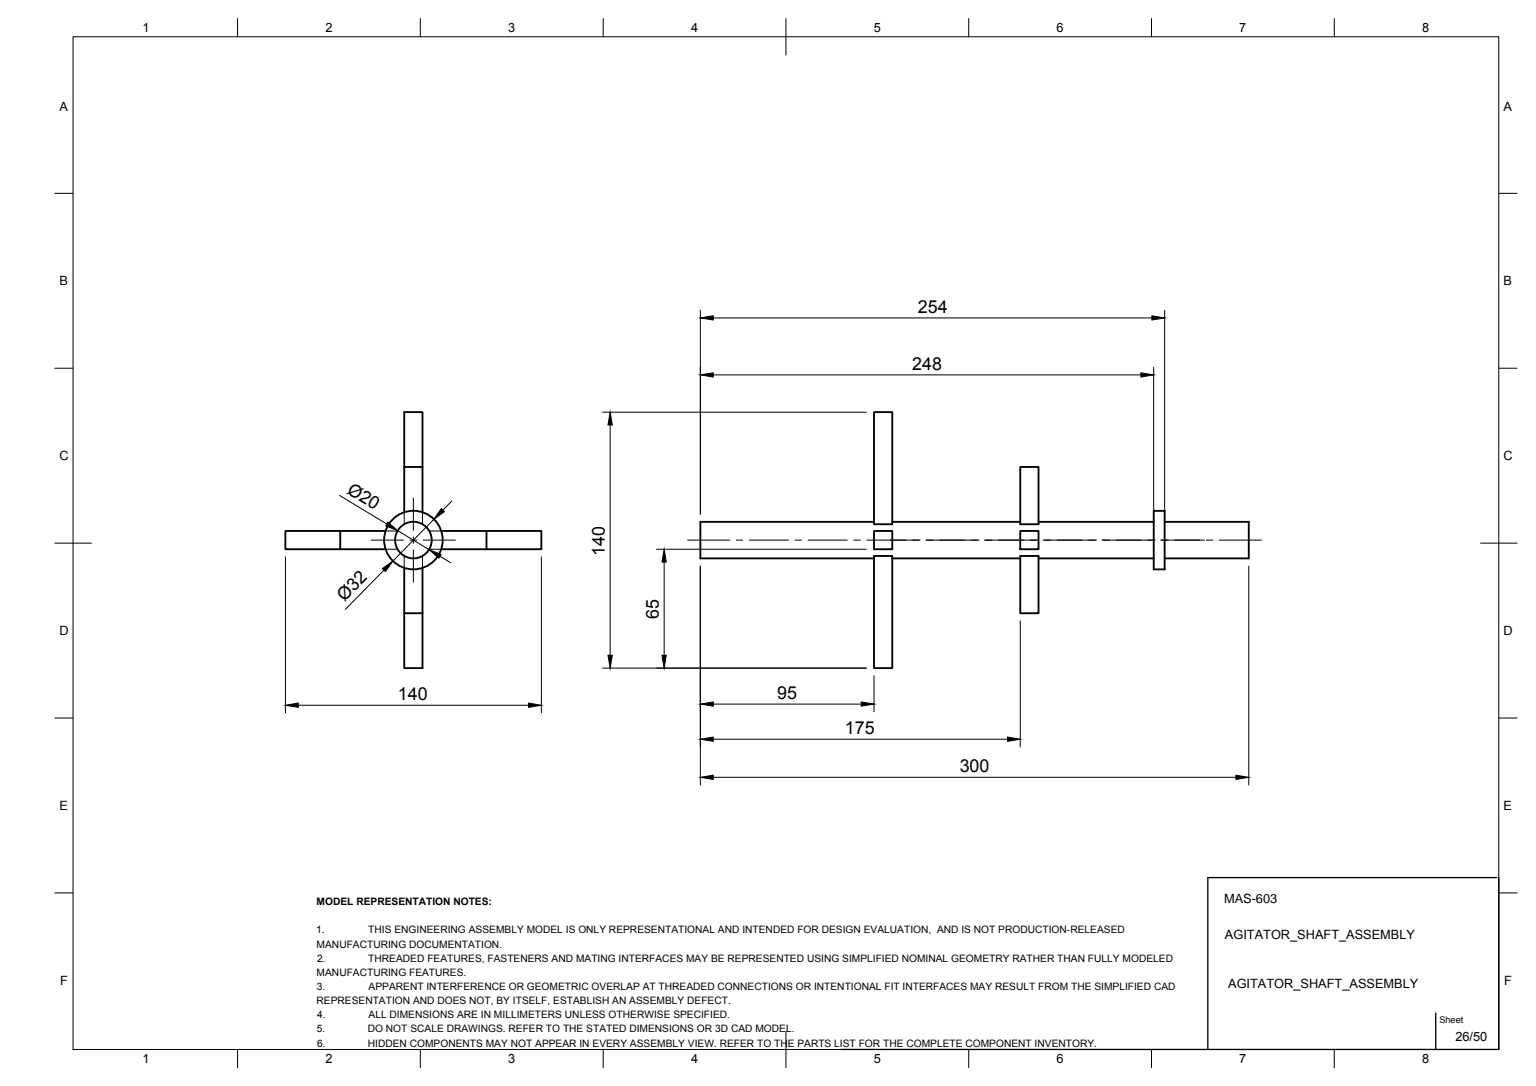
ISO-10303-21;
HEADER;
FILE_DESCRIPTION((''),'2;1');
FILE_NAME('AGITATOR_SHAFT_ASSEMBLY.step','2026-10-01T22:06:14-07:00',(''),(''),'','','');
FILE_SCHEMA (('AUTOMOTIVE_DESIGN { 1 0 10303 214 3 1 1 }'));
ENDSEC;
DATA;
#10=MECHANICAL_DESIGN_GEOMETRIC_PRESENTATION_REPRESENTATION('',(#1000),#50440);
#908=SHAPE_REPRESENTATION_RELATIONSHIP('SRR','None',#50640,#953) ;
#953=ADVANCED_BREP_SHAPE_REPRESENTATION('',(#1055),#50409) ;
#1000=STYLED_ITEM('',(#50889),#1055) ;
#1055=MANIFOLD_SOLID_BREP('AGITATOR_SHAFT_ASSEMBLY',#28667) ;
#1306=FACE_BOUND('',#4947,.T.) ;
#1307=FACE_BOUND('',#4949,.T.) ;
#1308=FACE_BOUND('',#4952,.T.) ;
#1309=FACE_BOUND('',#4953,.T.) ;
#1310=FACE_BOUND('',#4954,.T.) ;
#1311=FACE_BOUND('',#4955,.T.) ;
#1312=FACE_BOUND('',#4956,.T.) ;
#1313=FACE_BOUND('',#4957,.T.) ;
#2057=PLANE('',#30581) ;
#2058=PLANE('',#30584) ;
#2059=PLANE('',#30610) ;
#2060=PLANE('',#30611) ;
#2061=PLANE('',#30612) ;
#2062=PLANE('',#30613) ;
#2063=PLANE('',#30614) ;
#2064=PLANE('',#30615) ;
#2065=PLANE('',#30616) ;
#2066=PLANE('',#30617) ;
#2067=PLANE('',#30618) ;
#2068=PLANE('',#30619) ;
#2069=PLANE('',#30620) ;
#2070=PLANE('',#30621) ;
#2071=PLANE('',#30622) ;
#2072=PLANE('',#30623) ;
#2073=PLANE('',#30624) ;
#2074=PLANE('',#30625) ;
#2075=PLANE('',#30626) ;
#2076=PLANE('',#30627) ;
#2077=PLANE('',#30628) ;
#2078=PLANE('',#30629) ;
#2079=PLANE('',#30630) ;
#2080=PLANE('',#30631) ;
#2081=PLANE('',#30632) ;
#2082=PLANE('',#30633) ;
#2083=PLANE('',#30634) ;
#2084=PLANE('',#30635) ;
#2085=PLANE('',#30636) ;
#2086=PLANE('',#30637) ;
#2087=PLANE('',#30638) ;
#2088=PLANE('',#30639) ;
#2089=PLANE('',#30640) ;
#2090=PLANE('',#30641) ;
#2091=PLANE('',#30642) ;
#2092=PLANE('',#30643) ;
#2093=PLANE('',#30644) ;
#2094=PLANE('',#30645) ;
#2095=PLANE('',#30646) ;
#2096=PLANE('',#30647) ;
#2097=PLANE('',#30648) ;
#2098=PLANE('',#30649) ;
#2099=PLANE('',#30652) ;
#2100=PLANE('',#30653) ;
#3198=FACE_OUTER_BOUND('',#4946,.T.) ;
#3199=FACE_OUTER_BOUND('',#4948,.T.) ;
#3200=FACE_OUTER_BOUND('',#4950,.T.) ;
#3201=FACE_OUTER_BOUND('',#4951,.T.) ;
#3202=FACE_OUTER_BOUND('',#4958,.T.) ;
#3203=FACE_OUTER_BOUND('',#4959,.T.) ;
#3204=FACE_OUTER_BOUND('',#4960,.T.) ;
#3205=FACE_OUTER_BOUND('',#4961,.T.) ;
#3206=FACE_OUTER_BOUND('',#4962,.T.) ;
#3207=FACE_OUTER_BOUND('',#4963,.T.) ;
#3208=FACE_OUTER_BOUND('',#4964,.T.) ;
#3209=FACE_OUTER_BOUND('',#4965,.T.) ;
#3210=FACE_OUTER_BOUND('',#4966,.T.) ;
#3211=FACE_OUTER_BOUND('',#4967,.T.) ;
#3212=FACE_OUTER_BOUND('',#4968,.T.) ;
#3213=FACE_OUTER_BOUND('',#4969,.T.) ;
#3214=FACE_OUTER_BOUND('',#4970,.T.) ;
#3215=FACE_OUTER_BOUND('',#4971,.T.) ;
#3216=FACE_OUTER_BOUND('',#4972,.T.) ;
#3217=FACE_OUTER_BOUND('',#4973,.T.) ;
#3218=FACE_OUTER_BOUND('',#4974,.T.) ;
#3219=FACE_OUTER_BOUND('',#4975,.T.) ;
#3220=FACE_OUTER_BOUND('',#4976,.T.) ;
#3221=FACE_OUTER_BOUND('',#4977,.T.) ;
#3222=FACE_OUTER_BOUND('',#4978,.T.) ;
#3223=FACE_OUTER_BOUND('',#4979,.T.) ;
#3224=FACE_OUTER_BOUND('',#4980,.T.) ;
#3225=FACE_OUTER_BOUND('',#4981,.T.) ;
#3226=FACE_OUTER_BOUND('',#4982,.T.) ;
#3227=FACE_OUTER_BOUND('',#4983,.T.) ;
#3228=FACE_OUTER_BOUND('',#4984,.T.) ;
#3229=FACE_OUTER_BOUND('',#4985,.T.) ;
#3230=FACE_OUTER_BOUND('',#4986,.T.) ;
#3231=FACE_OUTER_BOUND('',#4987,.T.) ;
#3232=FACE_OUTER_BOUND('',#4988,.T.) ;
#3233=FACE_OUTER_BOUND('',#4989,.T.) ;
#3234=FACE_OUTER_BOUND('',#4990,.T.) ;
#3235=FACE_OUTER_BOUND('',#4991,.T.) ;
#3236=FACE_OUTER_BOUND('',#4992,.T.) ;
#3237=FACE_OUTER_BOUND('',#4993,.T.) ;
#3238=FACE_OUTER_BOUND('',#4994,.T.) ;
#3239=FACE_OUTER_BOUND('',#4995,.T.) ;
#3240=FACE_OUTER_BOUND('',#4996,.T.) ;
#3241=FACE_OUTER_BOUND('',#4997,.T.) ;
#3242=FACE_OUTER_BOUND('',#4998,.T.) ;
#3243=FACE_OUTER_BOUND('',#4999,.T.) ;
#3244=FACE_OUTER_BOUND('',#5000,.T.) ;
#4946=EDGE_LOOP('',(#23003)) ;
#4947=EDGE_LOOP('',(#23004)) ;
#4948=EDGE_LOOP('',(#23005)) ;
#4949=EDGE_LOOP('',(#23006)) ;
#4950=EDGE_LOOP('',(#23007,#23008,#23009,#23010)) ;
#4951=EDGE_LOOP('',(#23011,#23012,#23013,#23014,#23015,#23016,#23017,#23018,
#23019,#23020,#23021,#23022,#23023,#23024,#23025,#23026,#23027,#23028,#23029,
#23030)) ;
#4952=EDGE_LOOP('',(#23031,#23032,#23033,#23034)) ;
#4953=EDGE_LOOP('',(#23035,#23036,#23037,#23038)) ;
#4954=EDGE_LOOP('',(#23039,#23040,#23041,#23042)) ;
#4955=EDGE_LOOP('',(#23043,#23044,#23045,#23046)) ;
#4956=EDGE_LOOP('',(#23047,#23048,#23049,#23050)) ;
#4957=EDGE_LOOP('',(#23051,#23052,#23053,#23054)) ;
#4958=EDGE_LOOP('',(#23055,#23056,#23057,#23058)) ;
#4959=EDGE_LOOP('',(#23059,#23060,#23061,#23062)) ;
#4960=EDGE_LOOP('',(#23063,#23064,#23065,#23066)) ;
#4961=EDGE_LOOP('',(#23067,#23068,#23069,#23070)) ;
#4962=EDGE_LOOP('',(#23071,#23072,#23073,#23074)) ;
#4963=EDGE_LOOP('',(#23075,#23076,#23077,#23078)) ;
#4964=EDGE_LOOP('',(#23079,#23080,#23081,#23082)) ;
#4965=EDGE_LOOP('',(#23083,#23084,#23085,#23086)) ;
#4966=EDGE_LOOP('',(#23087,#23088,#23089,#23090)) ;
#4967=EDGE_LOOP('',(#23091,#23092,#23093,#23094)) ;
#4968=EDGE_LOOP('',(#23095,#23096,#23097,#23098)) ;
#4969=EDGE_LOOP('',(#23099,#23100,#23101,#23102)) ;
#4970=EDGE_LOOP('',(#23103,#23104,#23105,#23106)) ;
#4971=EDGE_LOOP('',(#23107,#23108,#23109,#23110,#23111)) ;
#4972=EDGE_LOOP('',(#23112,#23113,#23114,#23115)) ;
#4973=EDGE_LOOP('',(#23116,#23117,#23118,#23119)) ;
#4974=EDGE_LOOP('',(#23120,#23121,#23122,#23123)) ;
#4975=EDGE_LOOP('',(#23124,#23125,#23126,#23127,#23128)) ;
#4976=EDGE_LOOP('',(#23129,#23130,#23131,#23132)) ;
#4977=EDGE_LOOP('',(#23133,#23134,#23135,#23136)) ;
#4978=EDGE_LOOP('',(#23137,#23138,#23139,#23140)) ;
#4979=EDGE_LOOP('',(#23141,#23142,#23143,#23144)) ;
#4980=EDGE_LOOP('',(#23145,#23146,#23147,#23148)) ;
#4981=EDGE_LOOP('',(#23149,#23150,#23151,#23152)) ;
#4982=EDGE_LOOP('',(#23153,#23154,#23155,#23156)) ;
#4983=EDGE_LOOP('',(#23157,#23158,#23159,#23160)) ;
#4984=EDGE_LOOP('',(#23161,#23162,#23163,#23164)) ;
#4985=EDGE_LOOP('',(#23165,#23166,#23167,#23168)) ;
#4986=EDGE_LOOP('',(#23169,#23170,#23171,#23172)) ;
#4987=EDGE_LOOP('',(#23173,#23174,#23175,#23176)) ;
#4988=EDGE_LOOP('',(#23177,#23178,#23179,#23180)) ;
#4989=EDGE_LOOP('',(#23181,#23182,#23183,#23184)) ;
#4990=EDGE_LOOP('',(#23185,#23186,#23187,#23188)) ;
#4991=EDGE_LOOP('',(#23189,#23190,#23191,#23192,#23193)) ;
#4992=EDGE_LOOP('',(#23194,#23195,#23196,#23197)) ;
#4993=EDGE_LOOP('',(#23198,#23199,#23200,#23201)) ;
#4994=EDGE_LOOP('',(#23202,#23203,#23204,#23205)) ;
#4995=EDGE_LOOP('',(#23206,#23207,#23208,#23209,#23210)) ;
#4996=EDGE_LOOP('',(#23211,#23212,#23213,#23214)) ;
#4997=EDGE_LOOP('',(#23215,#23216,#23217,#23218)) ;
#4998=EDGE_LOOP('',(#23219,#23220,#23221,#23222)) ;
#4999=EDGE_LOOP('',(#23223)) ;
#5000=EDGE_LOOP('',(#23224)) ;
#7450=LINE('',#45964,#9922) ;
#7451=LINE('',#45969,#9923) ;
#7452=LINE('',#45973,#9924) ;
#7453=LINE('',#45977,#9925) ;
#7454=LINE('',#45981,#9926) ;
#7455=LINE('',#45984,#9927) ;
#7456=LINE('',#45988,#9928) ;
#7457=LINE('',#45993,#9929) ;
#7458=LINE('',#45997,#9930) ;
#7459=LINE('',#46001,#9931) ;
#7460=LINE('',#46005,#9932) ;
#7461=LINE('',#46009,#9933) ;
#7462=LINE('',#46013,#9934) ;
#7463=LINE('',#46017,#9935) ;
#7464=LINE('',#46021,#9936) ;
#7465=LINE('',#46025,#9937) ;
#7466=LINE('',#46029,#9938) ;
#7467=LINE('',#46033,#9939) ;
#7468=LINE('',#46037,#9940) ;
#7469=LINE('',#46041,#9941) ;
#7470=LINE('',#46045,#9942) ;
#7471=LINE('',#46047,#9943) ;
#7472=LINE('',#46048,#9944) ;
#7473=LINE('',#46051,#9945) ;
#7474=LINE('',#46052,#9946) ;
#7475=LINE('',#46055,#9947) ;
#7476=LINE('',#46056,#9948) ;
#7477=LINE('',#46059,#9949) ;
#7478=LINE('',#46061,#9950) ;
#7479=LINE('',#46062,#9951) ;
#7480=LINE('',#46064,#9952) ;
#7481=LINE('',#46067,#9953) ;
#7482=LINE('',#46068,#9954) ;
#7483=LINE('',#46071,#9955) ;
#7484=LINE('',#46072,#9956) ;
#7485=LINE('',#46075,#9957) ;
#7486=LINE('',#46079,#9958) ;
#7487=LINE('',#46081,#9959) ;
#7488=LINE('',#46082,#9960) ;
#7489=LINE('',#46085,#9961) ;
#7490=LINE('',#46086,#9962) ;
#7491=LINE('',#46089,#9963) ;
#7492=LINE('',#46090,#9964) ;
#7493=LINE('',#46093,#9965) ;
#7494=LINE('',#46095,#9966) ;
#7495=LINE('',#46096,#9967) ;
#7496=LINE('',#46098,#9968) ;
#7497=LINE('',#46101,#9969) ;
#7498=LINE('',#46102,#9970) ;
#7499=LINE('',#46105,#9971) ;
#7500=LINE('',#46106,#9972) ;
#7501=LINE('',#46108,#9973) ;
#7502=LINE('',#46113,#9974) ;
#7503=LINE('',#46115,#9975) ;
#7504=LINE('',#46116,#9976) ;
#7505=LINE('',#46119,#9977) ;
#7506=LINE('',#46120,#9978) ;
#7507=LINE('',#46123,#9979) ;
#7508=LINE('',#46124,#9980) ;
#7509=LINE('',#46127,#9981) ;
#7510=LINE('',#46129,#9982) ;
#7511=LINE('',#46130,#9983) ;
#7512=LINE('',#46132,#9984) ;
#7513=LINE('',#46135,#9985) ;
#7514=LINE('',#46136,#9986) ;
#7515=LINE('',#46139,#9987) ;
#7516=LINE('',#46140,#9988) ;
#7517=LINE('',#46143,#9989) ;
#7518=LINE('',#46147,#9990) ;
#7519=LINE('',#46149,#9991) ;
#7520=LINE('',#46150,#9992) ;
#7521=LINE('',#46153,#9993) ;
#7522=LINE('',#46154,#9994) ;
#7523=LINE('',#46157,#9995) ;
#7524=LINE('',#46158,#9996) ;
#7525=LINE('',#46161,#9997) ;
#7526=LINE('',#46163,#9998) ;
#7527=LINE('',#46164,#9999) ;
#7528=LINE('',#46166,#10000) ;
#7529=LINE('',#46169,#10001) ;
#7530=LINE('',#46170,#10002) ;
#7531=LINE('',#46173,#10003) ;
#7532=LINE('',#46174,#10004) ;
#7533=LINE('',#46176,#10005) ;
#7534=LINE('',#46181,#10006) ;
#9922=VECTOR('',#36851,1.6) ;
#9923=VECTOR('',#36856,1.) ;
#9924=VECTOR('',#36859,1.) ;
#9925=VECTOR('',#36862,1.) ;
#9926=VECTOR('',#36865,1.) ;
#9927=VECTOR('',#36868,1.) ;
#9928=VECTOR('',#36871,1.) ;
#9929=VECTOR('',#36876,1.) ;
#9930=VECTOR('',#36879,1.) ;
#9931=VECTOR('',#36882,1.) ;
#9932=VECTOR('',#36885,1.) ;
#9933=VECTOR('',#36888,1.) ;
#9934=VECTOR('',#36891,1.) ;
#9935=VECTOR('',#36894,1.) ;
#9936=VECTOR('',#36897,1.) ;
#9937=VECTOR('',#36900,1.) ;
#9938=VECTOR('',#36903,1.) ;
#9939=VECTOR('',#36906,1.) ;
#9940=VECTOR('',#36909,1.) ;
#9941=VECTOR('',#36912,1.) ;
#9942=VECTOR('',#36917,1.) ;
#9943=VECTOR('',#36918,1.) ;
#9944=VECTOR('',#36919,1.) ;
#9945=VECTOR('',#36922,1.) ;
#9946=VECTOR('',#36923,1.) ;
#9947=VECTOR('',#36926,1.) ;
#9948=VECTOR('',#36927,1.) ;
#9949=VECTOR('',#36930,1.) ;
#9950=VECTOR('',#36931,1.) ;
#9951=VECTOR('',#36932,1.) ;
#9952=VECTOR('',#36935,1.) ;
#9953=VECTOR('',#36938,1.) ;
#9954=VECTOR('',#36939,1.) ;
#9955=VECTOR('',#36942,1.) ;
#9956=VECTOR('',#36943,1.) ;
#9957=VECTOR('',#36948,1.) ;
#9958=VECTOR('',#36953,1.) ;
#9959=VECTOR('',#36954,1.) ;
#9960=VECTOR('',#36955,1.) ;
#9961=VECTOR('',#36958,1.) ;
#9962=VECTOR('',#36959,1.) ;
#9963=VECTOR('',#36962,1.) ;
#9964=VECTOR('',#36963,1.) ;
#9965=VECTOR('',#36966,1.) ;
#9966=VECTOR('',#36967,1.) ;
#9967=VECTOR('',#36968,1.) ;
#9968=VECTOR('',#36971,1.) ;
#9969=VECTOR('',#36974,1.) ;
#9970=VECTOR('',#36975,1.) ;
#9971=VECTOR('',#36978,1.) ;
#9972=VECTOR('',#36979,1.) ;
#9973=VECTOR('',#36982,1.) ;
#9974=VECTOR('',#36989,1.) ;
#9975=VECTOR('',#36990,1.) ;
#9976=VECTOR('',#36991,1.) ;
#9977=VECTOR('',#36994,1.) ;
#9978=VECTOR('',#36995,1.) ;
#9979=VECTOR('',#36998,1.) ;
#9980=VECTOR('',#36999,1.) ;
#9981=VECTOR('',#37002,1.) ;
#9982=VECTOR('',#37003,1.) ;
#9983=VECTOR('',#37004,1.) ;
#9984=VECTOR('',#37007,1.) ;
#9985=VECTOR('',#37010,1.) ;
#9986=VECTOR('',#37011,1.) ;
#9987=VECTOR('',#37014,1.) ;
#9988=VECTOR('',#37015,1.) ;
#9989=VECTOR('',#37020,1.) ;
#9990=VECTOR('',#37025,1.) ;
#9991=VECTOR('',#37026,1.) ;
#9992=VECTOR('',#37027,1.) ;
#9993=VECTOR('',#37030,1.) ;
#9994=VECTOR('',#37031,1.) ;
#9995=VECTOR('',#37034,1.) ;
#9996=VECTOR('',#37035,1.) ;
#9997=VECTOR('',#37038,1.) ;
#9998=VECTOR('',#37039,1.) ;
#9999=VECTOR('',#37040,1.) ;
#10000=VECTOR('',#37043,1.) ;
#10001=VECTOR('',#37046,1.) ;
#10002=VECTOR('',#37047,1.) ;
#10003=VECTOR('',#37050,1.) ;
#10004=VECTOR('',#37051,1.) ;
#10005=VECTOR('',#37054,1.) ;
#10006=VECTOR('',#37061,1.) ;
#11121=CIRCLE('',#30582,1.6) ;
#11122=CIRCLE('',#30583,1.) ;
#11123=CIRCLE('',#30585,1.6) ;
#11124=CIRCLE('',#30586,1.) ;
#11125=CIRCLE('',#30589,1.) ;
#11126=CIRCLE('',#30590,1.) ;
#11127=CIRCLE('',#30591,1.) ;
#11128=CIRCLE('',#30592,1.) ;
#11129=CIRCLE('',#30593,1.) ;
#11130=CIRCLE('',#30594,1.) ;
#11131=CIRCLE('',#30595,1.) ;
#11132=CIRCLE('',#30596,1.) ;
#11133=CIRCLE('',#30597,1.) ;
#11134=CIRCLE('',#30598,1.) ;
#11135=CIRCLE('',#30599,1.) ;
#11136=CIRCLE('',#30600,1.) ;
#11137=CIRCLE('',#30601,1.) ;
#11138=CIRCLE('',#30602,1.) ;
#11139=CIRCLE('',#30603,1.) ;
#11140=CIRCLE('',#30604,1.) ;
#11141=CIRCLE('',#30605,1.) ;
#11142=CIRCLE('',#30606,1.) ;
#11143=CIRCLE('',#30607,1.) ;
#11144=CIRCLE('',#30608,1.) ;
#11145=CIRCLE('',#30609,1.) ;
#11146=CIRCLE('',#30651,1.) ;
#13317=VERTEX_POINT('',#45954) ;
#13318=VERTEX_POINT('',#45956) ;
#13319=VERTEX_POINT('',#45959) ;
#13320=VERTEX_POINT('',#45961) ;
#13321=VERTEX_POINT('',#45966) ;
#13322=VERTEX_POINT('',#45968) ;
#13323=VERTEX_POINT('',#45970) ;
#13324=VERTEX_POINT('',#45972) ;
#13325=VERTEX_POINT('',#45974) ;
#13326=VERTEX_POINT('',#45976) ;
#13327=VERTEX_POINT('',#45978) ;
#13328=VERTEX_POINT('',#45980) ;
#13329=VERTEX_POINT('',#45982) ;
#13330=VERTEX_POINT('',#45985) ;
#13331=VERTEX_POINT('',#45987) ;
#13332=VERTEX_POINT('',#45990) ;
#13333=VERTEX_POINT('',#45992) ;
#13334=VERTEX_POINT('',#45995) ;
#13335=VERTEX_POINT('',#45996) ;
#13336=VERTEX_POINT('',#45998) ;
#13337=VERTEX_POINT('',#46000) ;
#13338=VERTEX_POINT('',#46003) ;
#13339=VERTEX_POINT('',#46004) ;
#13340=VERTEX_POINT('',#46006) ;
#13341=VERTEX_POINT('',#46008) ;
#13342=VERTEX_POINT('',#46011) ;
#13343=VERTEX_POINT('',#46012) ;
#13344=VERTEX_POINT('',#46014) ;
#13345=VERTEX_POINT('',#46016) ;
#13346=VERTEX_POINT('',#46019) ;
#13347=VERTEX_POINT('',#46020) ;
#13348=VERTEX_POINT('',#46022) ;
#13349=VERTEX_POINT('',#46024) ;
#13350=VERTEX_POINT('',#46027) ;
#13351=VERTEX_POINT('',#46028) ;
#13352=VERTEX_POINT('',#46030) ;
#13353=VERTEX_POINT('',#46032) ;
#13354=VERTEX_POINT('',#46035) ;
#13355=VERTEX_POINT('',#46036) ;
#13356=VERTEX_POINT('',#46038) ;
#13357=VERTEX_POINT('',#46040) ;
#13358=VERTEX_POINT('',#46044) ;
#13359=VERTEX_POINT('',#46046) ;
#13360=VERTEX_POINT('',#46050) ;
#13361=VERTEX_POINT('',#46054) ;
#13362=VERTEX_POINT('',#46058) ;
#13363=VERTEX_POINT('',#46060) ;
#13364=VERTEX_POINT('',#46066) ;
#13365=VERTEX_POINT('',#46070) ;
#13366=VERTEX_POINT('',#46078) ;
#13367=VERTEX_POINT('',#46080) ;
#13368=VERTEX_POINT('',#46084) ;
#13369=VERTEX_POINT('',#46088) ;
#13370=VERTEX_POINT('',#46092) ;
#13371=VERTEX_POINT('',#46094) ;
#13372=VERTEX_POINT('',#46100) ;
#13373=VERTEX_POINT('',#46104) ;
#13374=VERTEX_POINT('',#46112) ;
#13375=VERTEX_POINT('',#46114) ;
#13376=VERTEX_POINT('',#46118) ;
#13377=VERTEX_POINT('',#46122) ;
#13378=VERTEX_POINT('',#46126) ;
#13379=VERTEX_POINT('',#46128) ;
#13380=VERTEX_POINT('',#46134) ;
#13381=VERTEX_POINT('',#46138) ;
#13382=VERTEX_POINT('',#46146) ;
#13383=VERTEX_POINT('',#46148) ;
#13384=VERTEX_POINT('',#46152) ;
#13385=VERTEX_POINT('',#46156) ;
#13386=VERTEX_POINT('',#46160) ;
#13387=VERTEX_POINT('',#46162) ;
#13388=VERTEX_POINT('',#46168) ;
#13389=VERTEX_POINT('',#46172) ;
#13390=VERTEX_POINT('',#46180) ;
#16767=EDGE_CURVE('',#13317,#13317,#11121,.T.) ;
#16768=EDGE_CURVE('',#13318,#13318,#11122,.T.) ;
#16769=EDGE_CURVE('',#13319,#13319,#11123,.T.) ;
#16770=EDGE_CURVE('',#13320,#13320,#11124,.T.) ;
#16771=EDGE_CURVE('',#13319,#13317,#7450,.T.) ;
#16772=EDGE_CURVE('',#13321,#13321,#11125,.T.) ;
#16773=EDGE_CURVE('',#13321,#13322,#7451,.T.) ;
#16774=EDGE_CURVE('',#13322,#13323,#11126,.T.) ;
#16775=EDGE_CURVE('',#13323,#13324,#7452,.T.) ;
#16776=EDGE_CURVE('',#13324,#13325,#11127,.T.) ;
#16777=EDGE_CURVE('',#13325,#13326,#7453,.T.) ;
#16778=EDGE_CURVE('',#13326,#13327,#11128,.T.) ;
#16779=EDGE_CURVE('',#13327,#13328,#7454,.T.) ;
#16780=EDGE_CURVE('',#13328,#13329,#11129,.T.) ;
#16781=EDGE_CURVE('',#13329,#13320,#7455,.T.) ;
#16782=EDGE_CURVE('',#13329,#13330,#11130,.T.) ;
#16783=EDGE_CURVE('',#13330,#13331,#7456,.T.) ;
#16784=EDGE_CURVE('',#13331,#13326,#11131,.T.) ;
#16785=EDGE_CURVE('',#13325,#13332,#11132,.T.) ;
#16786=EDGE_CURVE('',#13332,#13333,#7457,.T.) ;
#16787=EDGE_CURVE('',#13333,#13322,#11133,.T.) ;
#16788=EDGE_CURVE('',#13334,#13335,#7458,.T.) ;
#16789=EDGE_CURVE('',#13335,#13336,#11134,.T.) ;
#16790=EDGE_CURVE('',#13336,#13337,#7459,.T.) ;
#16791=EDGE_CURVE('',#13337,#13334,#11135,.T.) ;
#16792=EDGE_CURVE('',#13338,#13339,#7460,.T.) ;
#16793=EDGE_CURVE('',#13339,#13340,#11136,.T.) ;
#16794=EDGE_CURVE('',#13340,#13341,#7461,.T.) ;
#16795=EDGE_CURVE('',#13341,#13338,#11137,.T.) ;
#16796=EDGE_CURVE('',#13342,#13343,#7462,.T.) ;
#16797=EDGE_CURVE('',#13343,#13344,#11138,.T.) ;
#16798=EDGE_CURVE('',#13344,#13345,#7463,.T.) ;
#16799=EDGE_CURVE('',#13345,#13342,#11139,.T.) ;
#16800=EDGE_CURVE('',#13346,#13347,#7464,.T.) ;
#16801=EDGE_CURVE('',#13347,#13348,#11140,.T.) ;
#16802=EDGE_CURVE('',#13348,#13349,#7465,.T.) ;
#16803=EDGE_CURVE('',#13349,#13346,#11141,.T.) ;
#16804=EDGE_CURVE('',#13350,#13351,#7466,.T.) ;
#16805=EDGE_CURVE('',#13351,#13352,#11142,.T.) ;
#16806=EDGE_CURVE('',#13352,#13353,#7467,.T.) ;
#16807=EDGE_CURVE('',#13353,#13350,#11143,.T.) ;
#16808=EDGE_CURVE('',#13354,#13355,#7468,.T.) ;
#16809=EDGE_CURVE('',#13355,#13356,#11144,.T.) ;
#16810=EDGE_CURVE('',#13356,#13357,#7469,.T.) ;
#16811=EDGE_CURVE('',#13357,#13354,#11145,.T.) ;
#16812=EDGE_CURVE('',#13352,#13358,#7470,.T.) ;
#16813=EDGE_CURVE('',#13358,#13359,#7471,.T.) ;
#16814=EDGE_CURVE('',#13359,#13353,#7472,.T.) ;
#16815=EDGE_CURVE('',#13360,#13351,#7473,.T.) ;
#16816=EDGE_CURVE('',#13358,#13360,#7474,.T.) ;
#16817=EDGE_CURVE('',#13359,#13361,#7475,.T.) ;
#16818=EDGE_CURVE('',#13350,#13361,#7476,.T.) ;
#16819=EDGE_CURVE('',#13362,#13355,#7477,.T.) ;
#16820=EDGE_CURVE('',#13363,#13362,#7478,.T.) ;
#16821=EDGE_CURVE('',#13356,#13363,#7479,.T.) ;
#16822=EDGE_CURVE('',#13361,#13360,#7480,.T.) ;
#16823=EDGE_CURVE('',#13354,#13364,#7481,.T.) ;
#16824=EDGE_CURVE('',#13364,#13362,#7482,.T.) ;
#16825=EDGE_CURVE('',#13363,#13365,#7483,.T.) ;
#16826=EDGE_CURVE('',#13365,#13357,#7484,.T.) ;
#16827=EDGE_CURVE('',#13365,#13364,#7485,.T.) ;
#16828=EDGE_CURVE('',#13348,#13366,#7486,.T.) ;
#16829=EDGE_CURVE('',#13366,#13367,#7487,.T.) ;
#16830=EDGE_CURVE('',#13367,#13349,#7488,.T.) ;
#16831=EDGE_CURVE('',#13368,#13347,#7489,.T.) ;
#16832=EDGE_CURVE('',#13366,#13368,#7490,.T.) ;
#16833=EDGE_CURVE('',#13367,#13369,#7491,.T.) ;
#16834=EDGE_CURVE('',#13346,#13369,#7492,.T.) ;
#16835=EDGE_CURVE('',#13370,#13333,#7493,.T.) ;
#16836=EDGE_CURVE('',#13371,#13370,#7494,.T.) ;
#16837=EDGE_CURVE('',#13323,#13371,#7495,.T.) ;
#16838=EDGE_CURVE('',#13369,#13368,#7496,.T.) ;
#16839=EDGE_CURVE('',#13332,#13372,#7497,.T.) ;
#16840=EDGE_CURVE('',#13372,#13370,#7498,.T.) ;
#16841=EDGE_CURVE('',#13371,#13373,#7499,.T.) ;
#16842=EDGE_CURVE('',#13373,#13324,#7500,.T.) ;
#16843=EDGE_CURVE('',#13373,#13372,#7501,.T.) ;
#16844=EDGE_CURVE('',#13340,#13374,#7502,.T.) ;
#16845=EDGE_CURVE('',#13374,#13375,#7503,.T.) ;
#16846=EDGE_CURVE('',#13375,#13341,#7504,.T.) ;
#16847=EDGE_CURVE('',#13376,#13339,#7505,.T.) ;
#16848=EDGE_CURVE('',#13374,#13376,#7506,.T.) ;
#16849=EDGE_CURVE('',#13375,#13377,#7507,.T.) ;
#16850=EDGE_CURVE('',#13338,#13377,#7508,.T.) ;
#16851=EDGE_CURVE('',#13378,#13343,#7509,.T.) ;
#16852=EDGE_CURVE('',#13379,#13378,#7510,.T.) ;
#16853=EDGE_CURVE('',#13344,#13379,#7511,.T.) ;
#16854=EDGE_CURVE('',#13377,#13376,#7512,.T.) ;
#16855=EDGE_CURVE('',#13342,#13380,#7513,.T.) ;
#16856=EDGE_CURVE('',#13380,#13378,#7514,.T.) ;
#16857=EDGE_CURVE('',#13379,#13381,#7515,.T.) ;
#16858=EDGE_CURVE('',#13381,#13345,#7516,.T.) ;
#16859=EDGE_CURVE('',#13381,#13380,#7517,.T.) ;
#16860=EDGE_CURVE('',#13336,#13382,#7518,.T.) ;
#16861=EDGE_CURVE('',#13382,#13383,#7519,.T.) ;
#16862=EDGE_CURVE('',#13383,#13337,#7520,.T.) ;
#16863=EDGE_CURVE('',#13384,#13335,#7521,.T.) ;
#16864=EDGE_CURVE('',#13382,#13384,#7522,.T.) ;
#16865=EDGE_CURVE('',#13383,#13385,#7523,.T.) ;
#16866=EDGE_CURVE('',#13334,#13385,#7524,.T.) ;
#16867=EDGE_CURVE('',#13386,#13331,#7525,.T.) ;
#16868=EDGE_CURVE('',#13387,#13386,#7526,.T.) ;
#16869=EDGE_CURVE('',#13327,#13387,#7527,.T.) ;
#16870=EDGE_CURVE('',#13385,#13384,#7528,.T.) ;
#16871=EDGE_CURVE('',#13330,#13388,#7529,.T.) ;
#16872=EDGE_CURVE('',#13388,#13386,#7530,.T.) ;
#16873=EDGE_CURVE('',#13387,#13389,#7531,.T.) ;
#16874=EDGE_CURVE('',#13389,#13328,#7532,.T.) ;
#16875=EDGE_CURVE('',#13389,#13388,#7533,.T.) ;
#16876=EDGE_CURVE('',#13318,#13390,#7534,.T.) ;
#16877=EDGE_CURVE('',#13390,#13390,#11146,.T.) ;
#23003=ORIENTED_EDGE('',*,*,#16767,.T.) ;
#23004=ORIENTED_EDGE('',*,*,#16768,.F.) ;
#23005=ORIENTED_EDGE('',*,*,#16769,.T.) ;
#23006=ORIENTED_EDGE('',*,*,#16770,.F.) ;
#23007=ORIENTED_EDGE('',*,*,#16769,.F.) ;
#23008=ORIENTED_EDGE('',*,*,#16771,.T.) ;
#23009=ORIENTED_EDGE('',*,*,#16767,.F.) ;
#23010=ORIENTED_EDGE('',*,*,#16771,.F.) ;
#23011=ORIENTED_EDGE('',*,*,#16772,.F.) ;
#23012=ORIENTED_EDGE('',*,*,#16773,.T.) ;
#23013=ORIENTED_EDGE('',*,*,#16774,.T.) ;
#23014=ORIENTED_EDGE('',*,*,#16775,.T.) ;
#23015=ORIENTED_EDGE('',*,*,#16776,.T.) ;
#23016=ORIENTED_EDGE('',*,*,#16777,.T.) ;
#23017=ORIENTED_EDGE('',*,*,#16778,.T.) ;
#23018=ORIENTED_EDGE('',*,*,#16779,.T.) ;
#23019=ORIENTED_EDGE('',*,*,#16780,.T.) ;
#23020=ORIENTED_EDGE('',*,*,#16781,.T.) ;
#23021=ORIENTED_EDGE('',*,*,#16770,.T.) ;
#23022=ORIENTED_EDGE('',*,*,#16781,.F.) ;
#23023=ORIENTED_EDGE('',*,*,#16782,.T.) ;
#23024=ORIENTED_EDGE('',*,*,#16783,.T.) ;
#23025=ORIENTED_EDGE('',*,*,#16784,.T.) ;
#23026=ORIENTED_EDGE('',*,*,#16777,.F.) ;
#23027=ORIENTED_EDGE('',*,*,#16785,.T.) ;
#23028=ORIENTED_EDGE('',*,*,#16786,.T.) ;
#23029=ORIENTED_EDGE('',*,*,#16787,.T.) ;
#23030=ORIENTED_EDGE('',*,*,#16773,.F.) ;
#23031=ORIENTED_EDGE('',*,*,#16788,.T.) ;
#23032=ORIENTED_EDGE('',*,*,#16789,.T.) ;
#23033=ORIENTED_EDGE('',*,*,#16790,.T.) ;
#23034=ORIENTED_EDGE('',*,*,#16791,.T.) ;
#23035=ORIENTED_EDGE('',*,*,#16792,.T.) ;
#23036=ORIENTED_EDGE('',*,*,#16793,.T.) ;
#23037=ORIENTED_EDGE('',*,*,#16794,.T.) ;
#23038=ORIENTED_EDGE('',*,*,#16795,.T.) ;
#23039=ORIENTED_EDGE('',*,*,#16796,.T.) ;
#23040=ORIENTED_EDGE('',*,*,#16797,.T.) ;
#23041=ORIENTED_EDGE('',*,*,#16798,.T.) ;
#23042=ORIENTED_EDGE('',*,*,#16799,.T.) ;
#23043=ORIENTED_EDGE('',*,*,#16800,.T.) ;
#23044=ORIENTED_EDGE('',*,*,#16801,.T.) ;
#23045=ORIENTED_EDGE('',*,*,#16802,.T.) ;
#23046=ORIENTED_EDGE('',*,*,#16803,.T.) ;
#23047=ORIENTED_EDGE('',*,*,#16804,.T.) ;
#23048=ORIENTED_EDGE('',*,*,#16805,.T.) ;
#23049=ORIENTED_EDGE('',*,*,#16806,.T.) ;
#23050=ORIENTED_EDGE('',*,*,#16807,.T.) ;
#23051=ORIENTED_EDGE('',*,*,#16808,.T.) ;
#23052=ORIENTED_EDGE('',*,*,#16809,.T.) ;
#23053=ORIENTED_EDGE('',*,*,#16810,.T.) ;
#23054=ORIENTED_EDGE('',*,*,#16811,.T.) ;
#23055=ORIENTED_EDGE('',*,*,#16806,.F.) ;
#23056=ORIENTED_EDGE('',*,*,#16812,.T.) ;
#23057=ORIENTED_EDGE('',*,*,#16813,.T.) ;
#23058=ORIENTED_EDGE('',*,*,#16814,.T.) ;
#23059=ORIENTED_EDGE('',*,*,#16805,.F.) ;
#23060=ORIENTED_EDGE('',*,*,#16815,.F.) ;
#23061=ORIENTED_EDGE('',*,*,#16816,.F.) ;
#23062=ORIENTED_EDGE('',*,*,#16812,.F.) ;
#23063=ORIENTED_EDGE('',*,*,#16807,.F.) ;
#23064=ORIENTED_EDGE('',*,*,#16814,.F.) ;
#23065=ORIENTED_EDGE('',*,*,#16817,.T.) ;
#23066=ORIENTED_EDGE('',*,*,#16818,.F.) ;
#23067=ORIENTED_EDGE('',*,*,#16809,.F.) ;
#23068=ORIENTED_EDGE('',*,*,#16819,.F.) ;
#23069=ORIENTED_EDGE('',*,*,#16820,.F.) ;
#23070=ORIENTED_EDGE('',*,*,#16821,.F.) ;
#23071=ORIENTED_EDGE('',*,*,#16804,.F.) ;
#23072=ORIENTED_EDGE('',*,*,#16818,.T.) ;
#23073=ORIENTED_EDGE('',*,*,#16822,.T.) ;
#23074=ORIENTED_EDGE('',*,*,#16815,.T.) ;
#23075=ORIENTED_EDGE('',*,*,#16808,.F.) ;
#23076=ORIENTED_EDGE('',*,*,#16823,.T.) ;
#23077=ORIENTED_EDGE('',*,*,#16824,.T.) ;
#23078=ORIENTED_EDGE('',*,*,#16819,.T.) ;
#23079=ORIENTED_EDGE('',*,*,#16810,.F.) ;
#23080=ORIENTED_EDGE('',*,*,#16821,.T.) ;
#23081=ORIENTED_EDGE('',*,*,#16825,.T.) ;
#23082=ORIENTED_EDGE('',*,*,#16826,.T.) ;
#23083=ORIENTED_EDGE('',*,*,#16816,.T.) ;
#23084=ORIENTED_EDGE('',*,*,#16822,.F.) ;
#23085=ORIENTED_EDGE('',*,*,#16817,.F.) ;
#23086=ORIENTED_EDGE('',*,*,#16813,.F.) ;
#23087=ORIENTED_EDGE('',*,*,#16811,.F.) ;
#23088=ORIENTED_EDGE('',*,*,#16826,.F.) ;
#23089=ORIENTED_EDGE('',*,*,#16827,.T.) ;
#23090=ORIENTED_EDGE('',*,*,#16823,.F.) ;
#23091=ORIENTED_EDGE('',*,*,#16820,.T.) ;
#23092=ORIENTED_EDGE('',*,*,#16824,.F.) ;
#23093=ORIENTED_EDGE('',*,*,#16827,.F.) ;
#23094=ORIENTED_EDGE('',*,*,#16825,.F.) ;
#23095=ORIENTED_EDGE('',*,*,#16802,.F.) ;
#23096=ORIENTED_EDGE('',*,*,#16828,.T.) ;
#23097=ORIENTED_EDGE('',*,*,#16829,.T.) ;
#23098=ORIENTED_EDGE('',*,*,#16830,.T.) ;
#23099=ORIENTED_EDGE('',*,*,#16801,.F.) ;
#23100=ORIENTED_EDGE('',*,*,#16831,.F.) ;
#23101=ORIENTED_EDGE('',*,*,#16832,.F.) ;
#23102=ORIENTED_EDGE('',*,*,#16828,.F.) ;
#23103=ORIENTED_EDGE('',*,*,#16803,.F.) ;
#23104=ORIENTED_EDGE('',*,*,#16830,.F.) ;
#23105=ORIENTED_EDGE('',*,*,#16833,.T.) ;
#23106=ORIENTED_EDGE('',*,*,#16834,.F.) ;
#23107=ORIENTED_EDGE('',*,*,#16787,.F.) ;
#23108=ORIENTED_EDGE('',*,*,#16835,.F.) ;
#23109=ORIENTED_EDGE('',*,*,#16836,.F.) ;
#23110=ORIENTED_EDGE('',*,*,#16837,.F.) ;
#23111=ORIENTED_EDGE('',*,*,#16774,.F.) ;
#23112=ORIENTED_EDGE('',*,*,#16800,.F.) ;
#23113=ORIENTED_EDGE('',*,*,#16834,.T.) ;
#23114=ORIENTED_EDGE('',*,*,#16838,.T.) ;
#23115=ORIENTED_EDGE('',*,*,#16831,.T.) ;
#23116=ORIENTED_EDGE('',*,*,#16786,.F.) ;
#23117=ORIENTED_EDGE('',*,*,#16839,.T.) ;
#23118=ORIENTED_EDGE('',*,*,#16840,.T.) ;
#23119=ORIENTED_EDGE('',*,*,#16835,.T.) ;
#23120=ORIENTED_EDGE('',*,*,#16775,.F.) ;
#23121=ORIENTED_EDGE('',*,*,#16837,.T.) ;
#23122=ORIENTED_EDGE('',*,*,#16841,.T.) ;
#23123=ORIENTED_EDGE('',*,*,#16842,.T.) ;
#23124=ORIENTED_EDGE('',*,*,#16776,.F.) ;
#23125=ORIENTED_EDGE('',*,*,#16842,.F.) ;
#23126=ORIENTED_EDGE('',*,*,#16843,.T.) ;
#23127=ORIENTED_EDGE('',*,*,#16839,.F.) ;
#23128=ORIENTED_EDGE('',*,*,#16785,.F.) ;
#23129=ORIENTED_EDGE('',*,*,#16836,.T.) ;
#23130=ORIENTED_EDGE('',*,*,#16840,.F.) ;
#23131=ORIENTED_EDGE('',*,*,#16843,.F.) ;
#23132=ORIENTED_EDGE('',*,*,#16841,.F.) ;
#23133=ORIENTED_EDGE('',*,*,#16832,.T.) ;
#23134=ORIENTED_EDGE('',*,*,#16838,.F.) ;
#23135=ORIENTED_EDGE('',*,*,#16833,.F.) ;
#23136=ORIENTED_EDGE('',*,*,#16829,.F.) ;
#23137=ORIENTED_EDGE('',*,*,#16794,.F.) ;
#23138=ORIENTED_EDGE('',*,*,#16844,.T.) ;
#23139=ORIENTED_EDGE('',*,*,#16845,.T.) ;
#23140=ORIENTED_EDGE('',*,*,#16846,.T.) ;
#23141=ORIENTED_EDGE('',*,*,#16793,.F.) ;
#23142=ORIENTED_EDGE('',*,*,#16847,.F.) ;
#23143=ORIENTED_EDGE('',*,*,#16848,.F.) ;
#23144=ORIENTED_EDGE('',*,*,#16844,.F.) ;
#23145=ORIENTED_EDGE('',*,*,#16795,.F.) ;
#23146=ORIENTED_EDGE('',*,*,#16846,.F.) ;
#23147=ORIENTED_EDGE('',*,*,#16849,.T.) ;
#23148=ORIENTED_EDGE('',*,*,#16850,.F.) ;
#23149=ORIENTED_EDGE('',*,*,#16797,.F.) ;
#23150=ORIENTED_EDGE('',*,*,#16851,.F.) ;
#23151=ORIENTED_EDGE('',*,*,#16852,.F.) ;
#23152=ORIENTED_EDGE('',*,*,#16853,.F.) ;
#23153=ORIENTED_EDGE('',*,*,#16792,.F.) ;
#23154=ORIENTED_EDGE('',*,*,#16850,.T.) ;
#23155=ORIENTED_EDGE('',*,*,#16854,.T.) ;
#23156=ORIENTED_EDGE('',*,*,#16847,.T.) ;
#23157=ORIENTED_EDGE('',*,*,#16796,.F.) ;
#23158=ORIENTED_EDGE('',*,*,#16855,.T.) ;
#23159=ORIENTED_EDGE('',*,*,#16856,.T.) ;
#23160=ORIENTED_EDGE('',*,*,#16851,.T.) ;
#23161=ORIENTED_EDGE('',*,*,#16798,.F.) ;
#23162=ORIENTED_EDGE('',*,*,#16853,.T.) ;
#23163=ORIENTED_EDGE('',*,*,#16857,.T.) ;
#23164=ORIENTED_EDGE('',*,*,#16858,.T.) ;
#23165=ORIENTED_EDGE('',*,*,#16848,.T.) ;
#23166=ORIENTED_EDGE('',*,*,#16854,.F.) ;
#23167=ORIENTED_EDGE('',*,*,#16849,.F.) ;
#23168=ORIENTED_EDGE('',*,*,#16845,.F.) ;
#23169=ORIENTED_EDGE('',*,*,#16799,.F.) ;
#23170=ORIENTED_EDGE('',*,*,#16858,.F.) ;
#23171=ORIENTED_EDGE('',*,*,#16859,.T.) ;
#23172=ORIENTED_EDGE('',*,*,#16855,.F.) ;
#23173=ORIENTED_EDGE('',*,*,#16852,.T.) ;
#23174=ORIENTED_EDGE('',*,*,#16856,.F.) ;
#23175=ORIENTED_EDGE('',*,*,#16859,.F.) ;
#23176=ORIENTED_EDGE('',*,*,#16857,.F.) ;
#23177=ORIENTED_EDGE('',*,*,#16790,.F.) ;
#23178=ORIENTED_EDGE('',*,*,#16860,.T.) ;
#23179=ORIENTED_EDGE('',*,*,#16861,.T.) ;
#23180=ORIENTED_EDGE('',*,*,#16862,.T.) ;
#23181=ORIENTED_EDGE('',*,*,#16789,.F.) ;
#23182=ORIENTED_EDGE('',*,*,#16863,.F.) ;
#23183=ORIENTED_EDGE('',*,*,#16864,.F.) ;
#23184=ORIENTED_EDGE('',*,*,#16860,.F.) ;
#23185=ORIENTED_EDGE('',*,*,#16791,.F.) ;
#23186=ORIENTED_EDGE('',*,*,#16862,.F.) ;
#23187=ORIENTED_EDGE('',*,*,#16865,.T.) ;
#23188=ORIENTED_EDGE('',*,*,#16866,.F.) ;
#23189=ORIENTED_EDGE('',*,*,#16784,.F.) ;
#23190=ORIENTED_EDGE('',*,*,#16867,.F.) ;
#23191=ORIENTED_EDGE('',*,*,#16868,.F.) ;
#23192=ORIENTED_EDGE('',*,*,#16869,.F.) ;
#23193=ORIENTED_EDGE('',*,*,#16778,.F.) ;
#23194=ORIENTED_EDGE('',*,*,#16788,.F.) ;
#23195=ORIENTED_EDGE('',*,*,#16866,.T.) ;
#23196=ORIENTED_EDGE('',*,*,#16870,.T.) ;
#23197=ORIENTED_EDGE('',*,*,#16863,.T.) ;
#23198=ORIENTED_EDGE('',*,*,#16783,.F.) ;
#23199=ORIENTED_EDGE('',*,*,#16871,.T.) ;
#23200=ORIENTED_EDGE('',*,*,#16872,.T.) ;
#23201=ORIENTED_EDGE('',*,*,#16867,.T.) ;
#23202=ORIENTED_EDGE('',*,*,#16779,.F.) ;
#23203=ORIENTED_EDGE('',*,*,#16869,.T.) ;
#23204=ORIENTED_EDGE('',*,*,#16873,.T.) ;
#23205=ORIENTED_EDGE('',*,*,#16874,.T.) ;
#23206=ORIENTED_EDGE('',*,*,#16780,.F.) ;
#23207=ORIENTED_EDGE('',*,*,#16874,.F.) ;
#23208=ORIENTED_EDGE('',*,*,#16875,.T.) ;
#23209=ORIENTED_EDGE('',*,*,#16871,.F.) ;
#23210=ORIENTED_EDGE('',*,*,#16782,.F.) ;
#23211=ORIENTED_EDGE('',*,*,#16868,.T.) ;
#23212=ORIENTED_EDGE('',*,*,#16872,.F.) ;
#23213=ORIENTED_EDGE('',*,*,#16875,.F.) ;
#23214=ORIENTED_EDGE('',*,*,#16873,.F.) ;
#23215=ORIENTED_EDGE('',*,*,#16864,.T.) ;
#23216=ORIENTED_EDGE('',*,*,#16870,.F.) ;
#23217=ORIENTED_EDGE('',*,*,#16865,.F.) ;
#23218=ORIENTED_EDGE('',*,*,#16861,.F.) ;
#23219=ORIENTED_EDGE('',*,*,#16768,.T.) ;
#23220=ORIENTED_EDGE('',*,*,#16876,.T.) ;
#23221=ORIENTED_EDGE('',*,*,#16877,.F.) ;
#23222=ORIENTED_EDGE('',*,*,#16876,.F.) ;
#23223=ORIENTED_EDGE('',*,*,#16877,.T.) ;
#23224=ORIENTED_EDGE('',*,*,#16772,.T.) ;
#26830=CYLINDRICAL_SURFACE('',#30587,1.6) ;
#26831=CYLINDRICAL_SURFACE('',#30588,1.) ;
#26832=CYLINDRICAL_SURFACE('',#30650,1.) ;
#27933=ADVANCED_FACE('',(#3198,#1306),#2057,.T.) ;
#27934=ADVANCED_FACE('',(#3199,#1307),#2058,.T.) ;
#27935=ADVANCED_FACE('',(#3200),#26830,.T.) ;
#27936=ADVANCED_FACE('',(#3201,#1308,#1309,#1310,#1311,#1312,#1313),#26831,
 .T.) ;
#27937=ADVANCED_FACE('',(#3202),#2059,.T.) ;
#27938=ADVANCED_FACE('',(#3203),#2060,.F.) ;
#27939=ADVANCED_FACE('',(#3204),#2061,.F.) ;
#27940=ADVANCED_FACE('',(#3205),#2062,.F.) ;
#27941=ADVANCED_FACE('',(#3206),#2063,.F.) ;
#27942=ADVANCED_FACE('',(#3207),#2064,.F.) ;
#27943=ADVANCED_FACE('',(#3208),#2065,.T.) ;
#27944=ADVANCED_FACE('',(#3209),#2066,.F.) ;
#27945=ADVANCED_FACE('',(#3210),#2067,.F.) ;
#27946=ADVANCED_FACE('',(#3211),#2068,.F.) ;
#27947=ADVANCED_FACE('',(#3212),#2069,.T.) ;
#27948=ADVANCED_FACE('',(#3213),#2070,.F.) ;
#27949=ADVANCED_FACE('',(#3214),#2071,.F.) ;
#27950=ADVANCED_FACE('',(#3215),#2072,.F.) ;
#27951=ADVANCED_FACE('',(#3216),#2073,.F.) ;
#27952=ADVANCED_FACE('',(#3217),#2074,.F.) ;
#27953=ADVANCED_FACE('',(#3218),#2075,.T.) ;
#27954=ADVANCED_FACE('',(#3219),#2076,.F.) ;
#27955=ADVANCED_FACE('',(#3220),#2077,.F.) ;
#27956=ADVANCED_FACE('',(#3221),#2078,.F.) ;
#27957=ADVANCED_FACE('',(#3222),#2079,.T.) ;
#27958=ADVANCED_FACE('',(#3223),#2080,.F.) ;
#27959=ADVANCED_FACE('',(#3224),#2081,.F.) ;
#27960=ADVANCED_FACE('',(#3225),#2082,.F.) ;
#27961=ADVANCED_FACE('',(#3226),#2083,.F.) ;
#27962=ADVANCED_FACE('',(#3227),#2084,.F.) ;
#27963=ADVANCED_FACE('',(#3228),#2085,.T.) ;
#27964=ADVANCED_FACE('',(#3229),#2086,.F.) ;
#27965=ADVANCED_FACE('',(#3230),#2087,.F.) ;
#27966=ADVANCED_FACE('',(#3231),#2088,.F.) ;
#27967=ADVANCED_FACE('',(#3232),#2089,.T.) ;
#27968=ADVANCED_FACE('',(#3233),#2090,.F.) ;
#27969=ADVANCED_FACE('',(#3234),#2091,.F.) ;
#27970=ADVANCED_FACE('',(#3235),#2092,.F.) ;
#27971=ADVANCED_FACE('',(#3236),#2093,.F.) ;
#27972=ADVANCED_FACE('',(#3237),#2094,.F.) ;
#27973=ADVANCED_FACE('',(#3238),#2095,.T.) ;
#27974=ADVANCED_FACE('',(#3239),#2096,.F.) ;
#27975=ADVANCED_FACE('',(#3240),#2097,.F.) ;
#27976=ADVANCED_FACE('',(#3241),#2098,.F.) ;
#27977=ADVANCED_FACE('',(#3242),#26832,.T.) ;
#27978=ADVANCED_FACE('',(#3243),#2099,.T.) ;
#27979=ADVANCED_FACE('',(#3244),#2100,.T.) ;
#28667=CLOSED_SHELL('',(#27933,#27934,#27935,#27936,#27937,#27938,#27939,
#27940,#27941,#27942,#27943,#27944,#27945,#27946,#27947,#27948,#27949,#27950,
#27951,#27952,#27953,#27954,#27955,#27956,#27957,#27958,#27959,#27960,#27961,
#27962,#27963,#27964,#27965,#27966,#27967,#27968,#27969,#27970,#27971,#27972,
#27973,#27974,#27975,#27976,#27977,#27978,#27979)) ;
#30580=AXIS2_PLACEMENT_3D('',#45952,#36835,#36836) ;
#30581=AXIS2_PLACEMENT_3D('',#45953,#36837,#36838) ;
#30582=AXIS2_PLACEMENT_3D('',#45955,#36839,#36840) ;
#30583=AXIS2_PLACEMENT_3D('',#45957,#36841,#36842) ;
#30584=AXIS2_PLACEMENT_3D('',#45958,#36843,#36844) ;
#30585=AXIS2_PLACEMENT_3D('',#45960,#36845,#36846) ;
#30586=AXIS2_PLACEMENT_3D('',#45962,#36847,#36848) ;
#30587=AXIS2_PLACEMENT_3D('',#45963,#36849,#36850) ;
#30588=AXIS2_PLACEMENT_3D('',#45965,#36852,#36853) ;
#30589=AXIS2_PLACEMENT_3D('',#45967,#36854,#36855) ;
#30590=AXIS2_PLACEMENT_3D('',#45971,#36857,#36858) ;
#30591=AXIS2_PLACEMENT_3D('',#45975,#36860,#36861) ;
#30592=AXIS2_PLACEMENT_3D('',#45979,#36863,#36864) ;
#30593=AXIS2_PLACEMENT_3D('',#45983,#36866,#36867) ;
#30594=AXIS2_PLACEMENT_3D('',#45986,#36869,#36870) ;
#30595=AXIS2_PLACEMENT_3D('',#45989,#36872,#36873) ;
#30596=AXIS2_PLACEMENT_3D('',#45991,#36874,#36875) ;
#30597=AXIS2_PLACEMENT_3D('',#45994,#36877,#36878) ;
#30598=AXIS2_PLACEMENT_3D('',#45999,#36880,#36881) ;
#30599=AXIS2_PLACEMENT_3D('',#46002,#36883,#36884) ;
#30600=AXIS2_PLACEMENT_3D('',#46007,#36886,#36887) ;
#30601=AXIS2_PLACEMENT_3D('',#46010,#36889,#36890) ;
#30602=AXIS2_PLACEMENT_3D('',#46015,#36892,#36893) ;
#30603=AXIS2_PLACEMENT_3D('',#46018,#36895,#36896) ;
#30604=AXIS2_PLACEMENT_3D('',#46023,#36898,#36899) ;
#30605=AXIS2_PLACEMENT_3D('',#46026,#36901,#36902) ;
#30606=AXIS2_PLACEMENT_3D('',#46031,#36904,#36905) ;
#30607=AXIS2_PLACEMENT_3D('',#46034,#36907,#36908) ;
#30608=AXIS2_PLACEMENT_3D('',#46039,#36910,#36911) ;
#30609=AXIS2_PLACEMENT_3D('',#46042,#36913,#36914) ;
#30610=AXIS2_PLACEMENT_3D('',#46043,#36915,#36916) ;
#30611=AXIS2_PLACEMENT_3D('',#46049,#36920,#36921) ;
#30612=AXIS2_PLACEMENT_3D('',#46053,#36924,#36925) ;
#30613=AXIS2_PLACEMENT_3D('',#46057,#36928,#36929) ;
#30614=AXIS2_PLACEMENT_3D('',#46063,#36933,#36934) ;
#30615=AXIS2_PLACEMENT_3D('',#46065,#36936,#36937) ;
#30616=AXIS2_PLACEMENT_3D('',#46069,#36940,#36941) ;
#30617=AXIS2_PLACEMENT_3D('',#46073,#36944,#36945) ;
#30618=AXIS2_PLACEMENT_3D('',#46074,#36946,#36947) ;
#30619=AXIS2_PLACEMENT_3D('',#46076,#36949,#36950) ;
#30620=AXIS2_PLACEMENT_3D('',#46077,#36951,#36952) ;
#30621=AXIS2_PLACEMENT_3D('',#46083,#36956,#36957) ;
#30622=AXIS2_PLACEMENT_3D('',#46087,#36960,#36961) ;
#30623=AXIS2_PLACEMENT_3D('',#46091,#36964,#36965) ;
#30624=AXIS2_PLACEMENT_3D('',#46097,#36969,#36970) ;
#30625=AXIS2_PLACEMENT_3D('',#46099,#36972,#36973) ;
#30626=AXIS2_PLACEMENT_3D('',#46103,#36976,#36977) ;
#30627=AXIS2_PLACEMENT_3D('',#46107,#36980,#36981) ;
#30628=AXIS2_PLACEMENT_3D('',#46109,#36983,#36984) ;
#30629=AXIS2_PLACEMENT_3D('',#46110,#36985,#36986) ;
#30630=AXIS2_PLACEMENT_3D('',#46111,#36987,#36988) ;
#30631=AXIS2_PLACEMENT_3D('',#46117,#36992,#36993) ;
#30632=AXIS2_PLACEMENT_3D('',#46121,#36996,#36997) ;
#30633=AXIS2_PLACEMENT_3D('',#46125,#37000,#37001) ;
#30634=AXIS2_PLACEMENT_3D('',#46131,#37005,#37006) ;
#30635=AXIS2_PLACEMENT_3D('',#46133,#37008,#37009) ;
#30636=AXIS2_PLACEMENT_3D('',#46137,#37012,#37013) ;
#30637=AXIS2_PLACEMENT_3D('',#46141,#37016,#37017) ;
#30638=AXIS2_PLACEMENT_3D('',#46142,#37018,#37019) ;
#30639=AXIS2_PLACEMENT_3D('',#46144,#37021,#37022) ;
#30640=AXIS2_PLACEMENT_3D('',#46145,#37023,#37024) ;
#30641=AXIS2_PLACEMENT_3D('',#46151,#37028,#37029) ;
#30642=AXIS2_PLACEMENT_3D('',#46155,#37032,#37033) ;
#30643=AXIS2_PLACEMENT_3D('',#46159,#37036,#37037) ;
#30644=AXIS2_PLACEMENT_3D('',#46165,#37041,#37042) ;
#30645=AXIS2_PLACEMENT_3D('',#46167,#37044,#37045) ;
#30646=AXIS2_PLACEMENT_3D('',#46171,#37048,#37049) ;
#30647=AXIS2_PLACEMENT_3D('',#46175,#37052,#37053) ;
#30648=AXIS2_PLACEMENT_3D('',#46177,#37055,#37056) ;
#30649=AXIS2_PLACEMENT_3D('',#46178,#37057,#37058) ;
#30650=AXIS2_PLACEMENT_3D('',#46179,#37059,#37060) ;
#30651=AXIS2_PLACEMENT_3D('',#46182,#37062,#37063) ;
#30652=AXIS2_PLACEMENT_3D('',#46183,#37064,#37065) ;
#30653=AXIS2_PLACEMENT_3D('',#46184,#37066,#37067) ;
#36835=DIRECTION('axis',(0.,0.,1.)) ;
#36836=DIRECTION('refdir',(1.,0.,0.)) ;
#36837=DIRECTION('center_axis',(0.,0.,-1.)) ;
#36838=DIRECTION('ref_axis',(-1.,0.,0.)) ;
#36839=DIRECTION('center_axis',(0.,0.,-1.)) ;
#36840=DIRECTION('ref_axis',(1.,0.,0.)) ;
#36841=DIRECTION('center_axis',(0.,0.,-1.)) ;
#36842=DIRECTION('ref_axis',(1.,0.,0.)) ;
#36843=DIRECTION('center_axis',(0.,0.,1.)) ;
#36844=DIRECTION('ref_axis',(1.,0.,0.)) ;
#36845=DIRECTION('center_axis',(0.,0.,1.)) ;
#36846=DIRECTION('ref_axis',(1.,0.,0.)) ;
#36847=DIRECTION('center_axis',(0.,0.,1.)) ;
#36848=DIRECTION('ref_axis',(1.,0.,0.)) ;
#36849=DIRECTION('center_axis',(0.,0.,1.)) ;
#36850=DIRECTION('ref_axis',(1.,0.,0.)) ;
#36851=DIRECTION('',(0.,0.,-1.)) ;
#36852=DIRECTION('center_axis',(0.,0.,1.)) ;
#36853=DIRECTION('ref_axis',(1.,0.,0.)) ;
#36854=DIRECTION('center_axis',(0.,0.,1.)) ;
#36855=DIRECTION('ref_axis',(1.,0.,0.)) ;
#36856=DIRECTION('',(0.,0.,-1.)) ;
#36857=DIRECTION('center_axis',(0.,0.,1.)) ;
#36858=DIRECTION('ref_axis',(1.,0.,0.)) ;
#36859=DIRECTION('',(0.,0.,-1.)) ;
#36860=DIRECTION('center_axis',(0.,0.,-1.)) ;
#36861=DIRECTION('ref_axis',(1.,0.,0.)) ;
#36862=DIRECTION('',(0.,0.,-1.)) ;
#36863=DIRECTION('center_axis',(0.,0.,1.)) ;
#36864=DIRECTION('ref_axis',(1.,0.,0.)) ;
#36865=DIRECTION('',(0.,0.,-1.)) ;
#36866=DIRECTION('center_axis',(0.,0.,-1.)) ;
#36867=DIRECTION('ref_axis',(1.,0.,0.)) ;
#36868=DIRECTION('',(0.,0.,-1.)) ;
#36869=DIRECTION('center_axis',(0.,0.,-1.)) ;
#36870=DIRECTION('ref_axis',(1.,0.,0.)) ;
#36871=DIRECTION('',(0.,0.,1.)) ;
#36872=DIRECTION('center_axis',(0.,0.,1.)) ;
#36873=DIRECTION('ref_axis',(1.,0.,0.)) ;
#36874=DIRECTION('center_axis',(0.,0.,-1.)) ;
#36875=DIRECTION('ref_axis',(1.,0.,0.)) ;
#36876=DIRECTION('',(0.,0.,1.)) ;
#36877=DIRECTION('center_axis',(0.,0.,1.)) ;
#36878=DIRECTION('ref_axis',(1.,0.,0.)) ;
#36879=DIRECTION('',(0.,0.,-1.)) ;
#36880=DIRECTION('center_axis',(0.,0.,-1.)) ;
#36881=DIRECTION('ref_axis',(1.,0.,0.)) ;
#36882=DIRECTION('',(0.,0.,1.)) ;
#36883=DIRECTION('center_axis',(0.,0.,1.)) ;
#36884=DIRECTION('ref_axis',(1.,0.,0.)) ;
#36885=DIRECTION('',(0.,0.,1.)) ;
#36886=DIRECTION('center_axis',(0.,0.,1.)) ;
#36887=DIRECTION('ref_axis',(1.,0.,0.)) ;
#36888=DIRECTION('',(0.,0.,-1.)) ;
#36889=DIRECTION('center_axis',(0.,0.,-1.)) ;
#36890=DIRECTION('ref_axis',(1.,0.,0.)) ;
#36891=DIRECTION('',(0.,0.,-1.)) ;
#36892=DIRECTION('center_axis',(0.,0.,-1.)) ;
#36893=DIRECTION('ref_axis',(1.,0.,0.)) ;
#36894=DIRECTION('',(0.,0.,1.)) ;
#36895=DIRECTION('center_axis',(0.,0.,1.)) ;
#36896=DIRECTION('ref_axis',(1.,0.,0.)) ;
#36897=DIRECTION('',(0.,0.,-1.)) ;
#36898=DIRECTION('center_axis',(0.,0.,-1.)) ;
#36899=DIRECTION('ref_axis',(1.,0.,0.)) ;
#36900=DIRECTION('',(0.,0.,1.)) ;
#36901=DIRECTION('center_axis',(0.,0.,1.)) ;
#36902=DIRECTION('ref_axis',(1.,0.,0.)) ;
#36903=DIRECTION('',(0.,0.,1.)) ;
#36904=DIRECTION('center_axis',(0.,0.,1.)) ;
#36905=DIRECTION('ref_axis',(1.,0.,0.)) ;
#36906=DIRECTION('',(0.,0.,-1.)) ;
#36907=DIRECTION('center_axis',(0.,0.,-1.)) ;
#36908=DIRECTION('ref_axis',(1.,0.,0.)) ;
#36909=DIRECTION('',(0.,0.,-1.)) ;
#36910=DIRECTION('center_axis',(0.,0.,-1.)) ;
#36911=DIRECTION('ref_axis',(1.,0.,0.)) ;
#36912=DIRECTION('',(0.,0.,1.)) ;
#36913=DIRECTION('center_axis',(0.,0.,1.)) ;
#36914=DIRECTION('ref_axis',(1.,0.,0.)) ;
#36915=DIRECTION('center_axis',(1.,-6.12323399573677E-17,0.)) ;
#36916=DIRECTION('ref_axis',(6.12323399573677E-17,1.,0.)) ;
#36917=DIRECTION('',(-6.12323399573677E-17,-1.,0.)) ;
#36918=DIRECTION('',(0.,0.,-1.)) ;
#36919=DIRECTION('',(6.12323399573677E-17,1.,0.)) ;
#36920=DIRECTION('center_axis',(0.,0.,-1.)) ;
#36921=DIRECTION('ref_axis',(-1.,6.12323399573677E-17,0.)) ;
#36922=DIRECTION('',(6.12323399573677E-17,1.,0.)) ;
#36923=DIRECTION('',(-1.,6.12323399573677E-17,0.)) ;
#36924=DIRECTION('center_axis',(0.,0.,1.)) ;
#36925=DIRECTION('ref_axis',(1.,-6.12323399573677E-17,0.)) ;
#36926=DIRECTION('',(-1.,6.12323399573677E-17,0.)) ;
#36927=DIRECTION('',(-6.12323399573677E-17,-1.,0.)) ;
#36928=DIRECTION('center_axis',(0.,0.,1.)) ;
#36929=DIRECTION('ref_axis',(1.,-6.12323399573677E-17,0.)) ;
#36930=DIRECTION('',(-6.12323399573677E-17,-1.,0.)) ;
#36931=DIRECTION('',(-1.,6.12323399573677E-17,0.)) ;
#36932=DIRECTION('',(6.12323399573677E-17,1.,0.)) ;
#36933=DIRECTION('center_axis',(1.,-6.12323399573677E-17,0.)) ;
#36934=DIRECTION('ref_axis',(6.12323399573677E-17,1.,0.)) ;
#36935=DIRECTION('',(0.,0.,1.)) ;
#36936=DIRECTION('center_axis',(1.,-6.12323399573677E-17,0.)) ;
#36937=DIRECTION('ref_axis',(6.12323399573677E-17,1.,0.)) ;
#36938=DIRECTION('',(6.12323399573677E-17,1.,0.)) ;
#36939=DIRECTION('',(0.,0.,-1.)) ;
#36940=DIRECTION('center_axis',(1.,-6.12323399573677E-17,0.)) ;
#36941=DIRECTION('ref_axis',(6.12323399573677E-17,1.,0.)) ;
#36942=DIRECTION('',(0.,0.,1.)) ;
#36943=DIRECTION('',(-6.12323399573677E-17,-1.,0.)) ;
#36944=DIRECTION('center_axis',(6.12323399573677E-17,1.,0.)) ;
#36945=DIRECTION('ref_axis',(-1.,6.12323399573677E-17,0.)) ;
#36946=DIRECTION('center_axis',(0.,0.,-1.)) ;
#36947=DIRECTION('ref_axis',(-1.,6.12323399573677E-17,0.)) ;
#36948=DIRECTION('',(-1.,6.12323399573677E-17,0.)) ;
#36949=DIRECTION('center_axis',(-6.12323399573677E-17,-1.,0.)) ;
#36950=DIRECTION('ref_axis',(1.,-6.12323399573677E-17,0.)) ;
#36951=DIRECTION('center_axis',(0.,-1.,0.)) ;
#36952=DIRECTION('ref_axis',(1.,0.,0.)) ;
#36953=DIRECTION('',(1.,0.,0.)) ;
#36954=DIRECTION('',(0.,0.,1.)) ;
#36955=DIRECTION('',(-1.,0.,0.)) ;
#36956=DIRECTION('center_axis',(0.,0.,1.)) ;
#36957=DIRECTION('ref_axis',(0.,-1.,0.)) ;
#36958=DIRECTION('',(-1.,0.,0.)) ;
#36959=DIRECTION('',(0.,1.,0.)) ;
#36960=DIRECTION('center_axis',(0.,0.,-1.)) ;
#36961=DIRECTION('ref_axis',(0.,1.,0.)) ;
#36962=DIRECTION('',(0.,1.,0.)) ;
#36963=DIRECTION('',(1.,0.,0.)) ;
#36964=DIRECTION('center_axis',(0.,0.,-1.)) ;
#36965=DIRECTION('ref_axis',(0.,1.,0.)) ;
#36966=DIRECTION('',(1.,0.,0.)) ;
#36967=DIRECTION('',(0.,1.,0.)) ;
#36968=DIRECTION('',(-1.,0.,0.)) ;
#36969=DIRECTION('center_axis',(0.,-1.,0.)) ;
#36970=DIRECTION('ref_axis',(1.,0.,0.)) ;
#36971=DIRECTION('',(0.,0.,-1.)) ;
#36972=DIRECTION('center_axis',(0.,-1.,0.)) ;
#36973=DIRECTION('ref_axis',(1.,0.,0.)) ;
#36974=DIRECTION('',(-1.,0.,0.)) ;
#36975=DIRECTION('',(0.,0.,1.)) ;
#36976=DIRECTION('center_axis',(0.,-1.,0.)) ;
#36977=DIRECTION('ref_axis',(1.,0.,0.)) ;
#36978=DIRECTION('',(0.,0.,-1.)) ;
#36979=DIRECTION('',(1.,0.,0.)) ;
#36980=DIRECTION('center_axis',(0.,0.,1.)) ;
#36981=DIRECTION('ref_axis',(0.,-1.,0.)) ;
#36982=DIRECTION('',(0.,1.,0.)) ;
#36983=DIRECTION('center_axis',(1.,0.,0.)) ;
#36984=DIRECTION('ref_axis',(0.,1.,0.)) ;
#36985=DIRECTION('center_axis',(-1.,0.,0.)) ;
#36986=DIRECTION('ref_axis',(0.,-1.,0.)) ;
#36987=DIRECTION('center_axis',(1.,-6.12323399573677E-17,0.)) ;
#36988=DIRECTION('ref_axis',(6.12323399573677E-17,1.,0.)) ;
#36989=DIRECTION('',(-6.12323399573677E-17,-1.,0.)) ;
#36990=DIRECTION('',(0.,0.,-1.)) ;
#36991=DIRECTION('',(6.12323399573677E-17,1.,0.)) ;
#36992=DIRECTION('center_axis',(0.,0.,-1.)) ;
#36993=DIRECTION('ref_axis',(-1.,6.12323399573677E-17,0.)) ;
#36994=DIRECTION('',(6.12323399573677E-17,1.,0.)) ;
#36995=DIRECTION('',(-1.,6.12323399573677E-17,0.)) ;
#36996=DIRECTION('center_axis',(0.,0.,1.)) ;
#36997=DIRECTION('ref_axis',(1.,-6.12323399573677E-17,0.)) ;
#36998=DIRECTION('',(-1.,6.12323399573677E-17,0.)) ;
#36999=DIRECTION('',(-6.12323399573677E-17,-1.,0.)) ;
#37000=DIRECTION('center_axis',(0.,0.,1.)) ;
#37001=DIRECTION('ref_axis',(1.,-6.12323399573677E-17,0.)) ;
#37002=DIRECTION('',(-6.12323399573677E-17,-1.,0.)) ;
#37003=DIRECTION('',(-1.,6.12323399573677E-17,0.)) ;
#37004=DIRECTION('',(6.12323399573677E-17,1.,0.)) ;
#37005=DIRECTION('center_axis',(1.,-6.12323399573677E-17,0.)) ;
#37006=DIRECTION('ref_axis',(6.12323399573677E-17,1.,0.)) ;
#37007=DIRECTION('',(0.,0.,1.)) ;
#37008=DIRECTION('center_axis',(1.,-6.12323399573677E-17,0.)) ;
#37009=DIRECTION('ref_axis',(6.12323399573677E-17,1.,0.)) ;
#37010=DIRECTION('',(6.12323399573677E-17,1.,0.)) ;
#37011=DIRECTION('',(0.,0.,-1.)) ;
#37012=DIRECTION('center_axis',(1.,-6.12323399573677E-17,0.)) ;
#37013=DIRECTION('ref_axis',(6.12323399573677E-17,1.,0.)) ;
#37014=DIRECTION('',(0.,0.,1.)) ;
#37015=DIRECTION('',(-6.12323399573677E-17,-1.,0.)) ;
#37016=DIRECTION('center_axis',(6.12323399573677E-17,1.,0.)) ;
#37017=DIRECTION('ref_axis',(-1.,6.12323399573677E-17,0.)) ;
#37018=DIRECTION('center_axis',(0.,0.,-1.)) ;
#37019=DIRECTION('ref_axis',(-1.,6.12323399573677E-17,0.)) ;
#37020=DIRECTION('',(-1.,6.12323399573677E-17,0.)) ;
#37021=DIRECTION('center_axis',(-6.12323399573677E-17,-1.,0.)) ;
#37022=DIRECTION('ref_axis',(1.,-6.12323399573677E-17,0.)) ;
#37023=DIRECTION('center_axis',(0.,-1.,0.)) ;
#37024=DIRECTION('ref_axis',(1.,0.,0.)) ;
#37025=DIRECTION('',(1.,0.,0.)) ;
#37026=DIRECTION('',(0.,0.,1.)) ;
#37027=DIRECTION('',(-1.,0.,0.)) ;
#37028=DIRECTION('center_axis',(0.,0.,1.)) ;
#37029=DIRECTION('ref_axis',(0.,-1.,0.)) ;
#37030=DIRECTION('',(-1.,0.,0.)) ;
#37031=DIRECTION('',(0.,1.,0.)) ;
#37032=DIRECTION('center_axis',(0.,0.,-1.)) ;
#37033=DIRECTION('ref_axis',(0.,1.,0.)) ;
#37034=DIRECTION('',(0.,1.,0.)) ;
#37035=DIRECTION('',(1.,0.,0.)) ;
#37036=DIRECTION('center_axis',(0.,0.,-1.)) ;
#37037=DIRECTION('ref_axis',(0.,1.,0.)) ;
#37038=DIRECTION('',(1.,0.,0.)) ;
#37039=DIRECTION('',(0.,1.,0.)) ;
#37040=DIRECTION('',(-1.,0.,0.)) ;
#37041=DIRECTION('center_axis',(0.,-1.,0.)) ;
#37042=DIRECTION('ref_axis',(1.,0.,0.)) ;
#37043=DIRECTION('',(0.,0.,-1.)) ;
#37044=DIRECTION('center_axis',(0.,-1.,0.)) ;
#37045=DIRECTION('ref_axis',(1.,0.,0.)) ;
#37046=DIRECTION('',(-1.,0.,0.)) ;
#37047=DIRECTION('',(0.,0.,1.)) ;
#37048=DIRECTION('center_axis',(0.,-1.,0.)) ;
#37049=DIRECTION('ref_axis',(1.,0.,0.)) ;
#37050=DIRECTION('',(0.,0.,-1.)) ;
#37051=DIRECTION('',(1.,0.,0.)) ;
#37052=DIRECTION('center_axis',(0.,0.,1.)) ;
#37053=DIRECTION('ref_axis',(0.,-1.,0.)) ;
#37054=DIRECTION('',(0.,1.,0.)) ;
#37055=DIRECTION('center_axis',(1.,0.,0.)) ;
#37056=DIRECTION('ref_axis',(0.,1.,0.)) ;
#37057=DIRECTION('center_axis',(-1.,0.,0.)) ;
#37058=DIRECTION('ref_axis',(0.,-1.,0.)) ;
#37059=DIRECTION('center_axis',(0.,0.,1.)) ;
#37060=DIRECTION('ref_axis',(1.,0.,0.)) ;
#37061=DIRECTION('',(0.,0.,-1.)) ;
#37062=DIRECTION('center_axis',(0.,0.,-1.)) ;
#37063=DIRECTION('ref_axis',(1.,0.,0.)) ;
#37064=DIRECTION('center_axis',(0.,0.,-1.)) ;
#37065=DIRECTION('ref_axis',(-1.,0.,0.)) ;
#37066=DIRECTION('center_axis',(0.,0.,1.)) ;
#37067=DIRECTION('ref_axis',(1.,0.,0.)) ;
#45952=CARTESIAN_POINT('',(0.,0.,0.)) ;
#45953=CARTESIAN_POINT('Origin',(0.,-8.5,44.6)) ;
#45954=CARTESIAN_POINT('',(-1.6,-8.5,44.6)) ;
#45955=CARTESIAN_POINT('Origin',(0.,-8.5,44.6)) ;
#45956=CARTESIAN_POINT('',(-1.,-8.5,44.6)) ;
#45957=CARTESIAN_POINT('Origin',(0.,-8.5,44.6)) ;
#45958=CARTESIAN_POINT('Origin',(0.,-8.5,45.2)) ;
#45959=CARTESIAN_POINT('',(-1.6,-8.5,45.2)) ;
#45960=CARTESIAN_POINT('Origin',(0.,-8.5,45.2)) ;
#45961=CARTESIAN_POINT('',(-1.,-8.5,45.2)) ;
#45962=CARTESIAN_POINT('Origin',(0.,-8.5,45.2)) ;
#45963=CARTESIAN_POINT('Origin',(0.,-8.5,44.9)) ;
#45964=CARTESIAN_POINT('',(-1.6,-8.5,44.9)) ;
#45965=CARTESIAN_POINT('Origin',(0.,-8.5,55.)) ;
#45966=CARTESIAN_POINT('',(-1.,-8.5,70.)) ;
#45967=CARTESIAN_POINT('Origin',(0.,-8.5,70.)) ;
#45968=CARTESIAN_POINT('',(-1.,-8.5,60.5)) ;
#45969=CARTESIAN_POINT('',(-1.,-8.5,55.)) ;
#45970=CARTESIAN_POINT('',(-0.866025403784439,-9.,60.5)) ;
#45971=CARTESIAN_POINT('Origin',(0.,-8.5,60.5)) ;
#45972=CARTESIAN_POINT('',(-0.866025403784439,-9.,59.5)) ;
#45973=CARTESIAN_POINT('',(-0.866025403784439,-9.,55.)) ;
#45974=CARTESIAN_POINT('',(-1.,-8.5,59.5)) ;
#45975=CARTESIAN_POINT('Origin',(0.,-8.5,59.5)) ;
#45976=CARTESIAN_POINT('',(-1.,-8.5,52.5)) ;
#45977=CARTESIAN_POINT('',(-1.,-8.5,55.)) ;
#45978=CARTESIAN_POINT('',(-0.866025403784439,-9.,52.5)) ;
#45979=CARTESIAN_POINT('Origin',(0.,-8.5,52.5)) ;
#45980=CARTESIAN_POINT('',(-0.866025403784439,-9.,51.5)) ;
#45981=CARTESIAN_POINT('',(-0.866025403784439,-9.,55.)) ;
#45982=CARTESIAN_POINT('',(-1.,-8.5,51.5)) ;
#45983=CARTESIAN_POINT('Origin',(0.,-8.5,51.5)) ;
#45984=CARTESIAN_POINT('',(-1.,-8.5,55.)) ;
#45985=CARTESIAN_POINT('',(-0.866025403784439,-8.,51.5)) ;
#45986=CARTESIAN_POINT('Origin',(0.,-8.5,51.5)) ;
#45987=CARTESIAN_POINT('',(-0.866025403784439,-8.,52.5)) ;
#45988=CARTESIAN_POINT('',(-0.866025403784439,-8.,55.)) ;
#45989=CARTESIAN_POINT('Origin',(0.,-8.5,52.5)) ;
#45990=CARTESIAN_POINT('',(-0.866025403784439,-8.,59.5)) ;
#45991=CARTESIAN_POINT('Origin',(0.,-8.5,59.5)) ;
#45992=CARTESIAN_POINT('',(-0.866025403784439,-8.,60.5)) ;
#45993=CARTESIAN_POINT('',(-0.866025403784439,-8.,55.)) ;
#45994=CARTESIAN_POINT('Origin',(0.,-8.5,60.5)) ;
#45995=CARTESIAN_POINT('',(0.866025403784439,-8.,52.5)) ;
#45996=CARTESIAN_POINT('',(0.866025403784439,-8.,51.5)) ;
#45997=CARTESIAN_POINT('',(0.866025403784439,-8.,55.)) ;
#45998=CARTESIAN_POINT('',(0.866025403784439,-9.,51.5)) ;
#45999=CARTESIAN_POINT('Origin',(0.,-8.5,51.5)) ;
#46000=CARTESIAN_POINT('',(0.866025403784439,-9.,52.5)) ;
#46001=CARTESIAN_POINT('',(0.866025403784439,-9.,55.)) ;
#46002=CARTESIAN_POINT('Origin',(0.,-8.5,52.5)) ;
#46003=CARTESIAN_POINT('',(-0.5,-9.36602540378444,51.5)) ;
#46004=CARTESIAN_POINT('',(-0.5,-9.36602540378444,52.5)) ;
#46005=CARTESIAN_POINT('',(-0.5,-9.36602540378444,55.)) ;
#46006=CARTESIAN_POINT('',(0.5,-9.36602540378444,52.5)) ;
#46007=CARTESIAN_POINT('Origin',(0.,-8.5,52.5)) ;
#46008=CARTESIAN_POINT('',(0.5,-9.36602540378444,51.5)) ;
#46009=CARTESIAN_POINT('',(0.5,-9.36602540378444,55.)) ;
#46010=CARTESIAN_POINT('Origin',(0.,-8.5,51.5)) ;
#46011=CARTESIAN_POINT('',(-0.5,-7.63397459621556,52.5)) ;
#46012=CARTESIAN_POINT('',(-0.5,-7.63397459621556,51.5)) ;
#46013=CARTESIAN_POINT('',(-0.5,-7.63397459621556,55.)) ;
#46014=CARTESIAN_POINT('',(0.5,-7.63397459621556,51.5)) ;
#46015=CARTESIAN_POINT('Origin',(0.,-8.5,51.5)) ;
#46016=CARTESIAN_POINT('',(0.5,-7.63397459621556,52.5)) ;
#46017=CARTESIAN_POINT('',(0.5,-7.63397459621556,55.)) ;
#46018=CARTESIAN_POINT('Origin',(0.,-8.5,52.5)) ;
#46019=CARTESIAN_POINT('',(0.866025403784439,-8.,60.5)) ;
#46020=CARTESIAN_POINT('',(0.866025403784439,-8.,59.5)) ;
#46021=CARTESIAN_POINT('',(0.866025403784439,-8.,55.)) ;
#46022=CARTESIAN_POINT('',(0.866025403784439,-9.,59.5)) ;
#46023=CARTESIAN_POINT('Origin',(0.,-8.5,59.5)) ;
#46024=CARTESIAN_POINT('',(0.866025403784439,-9.,60.5)) ;
#46025=CARTESIAN_POINT('',(0.866025403784439,-9.,55.)) ;
#46026=CARTESIAN_POINT('Origin',(0.,-8.5,60.5)) ;
#46027=CARTESIAN_POINT('',(-0.5,-9.36602540378444,59.5)) ;
#46028=CARTESIAN_POINT('',(-0.5,-9.36602540378444,60.5)) ;
#46029=CARTESIAN_POINT('',(-0.5,-9.36602540378444,55.)) ;
#46030=CARTESIAN_POINT('',(0.5,-9.36602540378444,60.5)) ;
#46031=CARTESIAN_POINT('Origin',(0.,-8.5,60.5)) ;
#46032=CARTESIAN_POINT('',(0.5,-9.36602540378444,59.5)) ;
#46033=CARTESIAN_POINT('',(0.5,-9.36602540378444,55.)) ;
#46034=CARTESIAN_POINT('Origin',(0.,-8.5,59.5)) ;
#46035=CARTESIAN_POINT('',(-0.5,-7.63397459621556,60.5)) ;
#46036=CARTESIAN_POINT('',(-0.5,-7.63397459621556,59.5)) ;
#46037=CARTESIAN_POINT('',(-0.5,-7.63397459621556,55.)) ;
#46038=CARTESIAN_POINT('',(0.5,-7.63397459621556,59.5)) ;
#46039=CARTESIAN_POINT('Origin',(0.,-8.5,59.5)) ;
#46040=CARTESIAN_POINT('',(0.5,-7.63397459621556,60.5)) ;
#46041=CARTESIAN_POINT('',(0.5,-7.63397459621556,55.)) ;
#46042=CARTESIAN_POINT('Origin',(0.,-8.5,60.5)) ;
#46043=CARTESIAN_POINT('Origin',(0.5,-8.5,60.)) ;
#46044=CARTESIAN_POINT('',(0.5,-15.5,60.5)) ;
#46045=CARTESIAN_POINT('',(0.5,-8.5,60.5)) ;
#46046=CARTESIAN_POINT('',(0.5,-15.5,59.5)) ;
#46047=CARTESIAN_POINT('',(0.5,-15.5,60.)) ;
#46048=CARTESIAN_POINT('',(0.5,-8.5,59.5)) ;
#46049=CARTESIAN_POINT('Origin',(0.,-8.5,60.5)) ;
#46050=CARTESIAN_POINT('',(-0.5,-15.5,60.5)) ;
#46051=CARTESIAN_POINT('',(-0.5,-8.5,60.5)) ;
#46052=CARTESIAN_POINT('',(-4.28626379701574E-16,-15.5,60.5)) ;
#46053=CARTESIAN_POINT('Origin',(0.,-8.5,59.5)) ;
#46054=CARTESIAN_POINT('',(-0.5,-15.5,59.5)) ;
#46055=CARTESIAN_POINT('',(-4.28626379701574E-16,-15.5,59.5)) ;
#46056=CARTESIAN_POINT('',(-0.5,-8.5,59.5)) ;
#46057=CARTESIAN_POINT('Origin',(0.,-8.5,59.5)) ;
#46058=CARTESIAN_POINT('',(-0.5,-1.5,59.5)) ;
#46059=CARTESIAN_POINT('',(-0.5,-8.5,59.5)) ;
#46060=CARTESIAN_POINT('',(0.5,-1.5,59.5)) ;
#46061=CARTESIAN_POINT('',(4.28626379701574E-16,-1.5,59.5)) ;
#46062=CARTESIAN_POINT('',(0.5,-8.5,59.5)) ;
#46063=CARTESIAN_POINT('Origin',(-0.5,-8.5,60.)) ;
#46064=CARTESIAN_POINT('',(-0.5,-15.5,60.)) ;
#46065=CARTESIAN_POINT('Origin',(-0.5,-8.5,60.)) ;
#46066=CARTESIAN_POINT('',(-0.5,-1.5,60.5)) ;
#46067=CARTESIAN_POINT('',(-0.5,-8.5,60.5)) ;
#46068=CARTESIAN_POINT('',(-0.5,-1.5,60.)) ;
#46069=CARTESIAN_POINT('Origin',(0.5,-8.5,60.)) ;
#46070=CARTESIAN_POINT('',(0.5,-1.5,60.5)) ;
#46071=CARTESIAN_POINT('',(0.5,-1.5,60.)) ;
#46072=CARTESIAN_POINT('',(0.5,-8.5,60.5)) ;
#46073=CARTESIAN_POINT('Origin',(-4.28626379701574E-16,-15.5,60.)) ;
#46074=CARTESIAN_POINT('Origin',(0.,-8.5,60.5)) ;
#46075=CARTESIAN_POINT('',(4.28626379701574E-16,-1.5,60.5)) ;
#46076=CARTESIAN_POINT('Origin',(4.28626379701574E-16,-1.5,60.)) ;
#46077=CARTESIAN_POINT('Origin',(0.,-9.,60.)) ;
#46078=CARTESIAN_POINT('',(7.,-9.,59.5)) ;
#46079=CARTESIAN_POINT('',(0.,-9.,59.5)) ;
#46080=CARTESIAN_POINT('',(7.,-9.,60.5)) ;
#46081=CARTESIAN_POINT('',(7.,-9.,60.)) ;
#46082=CARTESIAN_POINT('',(0.,-9.,60.5)) ;
#46083=CARTESIAN_POINT('Origin',(0.,-8.5,59.5)) ;
#46084=CARTESIAN_POINT('',(7.,-8.,59.5)) ;
#46085=CARTESIAN_POINT('',(0.,-8.,59.5)) ;
#46086=CARTESIAN_POINT('',(7.,-8.5,59.5)) ;
#46087=CARTESIAN_POINT('Origin',(0.,-8.5,60.5)) ;
#46088=CARTESIAN_POINT('',(7.,-8.,60.5)) ;
#46089=CARTESIAN_POINT('',(7.,-8.5,60.5)) ;
#46090=CARTESIAN_POINT('',(0.,-8.,60.5)) ;
#46091=CARTESIAN_POINT('Origin',(0.,-8.5,60.5)) ;
#46092=CARTESIAN_POINT('',(-7.,-8.,60.5)) ;
#46093=CARTESIAN_POINT('',(0.,-8.,60.5)) ;
#46094=CARTESIAN_POINT('',(-7.,-9.,60.5)) ;
#46095=CARTESIAN_POINT('',(-7.,-8.5,60.5)) ;
#46096=CARTESIAN_POINT('',(0.,-9.,60.5)) ;
#46097=CARTESIAN_POINT('Origin',(0.,-8.,60.)) ;
#46098=CARTESIAN_POINT('',(7.,-8.,60.)) ;
#46099=CARTESIAN_POINT('Origin',(0.,-8.,60.)) ;
#46100=CARTESIAN_POINT('',(-7.,-8.,59.5)) ;
#46101=CARTESIAN_POINT('',(0.,-8.,59.5)) ;
#46102=CARTESIAN_POINT('',(-7.,-8.,60.)) ;
#46103=CARTESIAN_POINT('Origin',(0.,-9.,60.)) ;
#46104=CARTESIAN_POINT('',(-7.,-9.,59.5)) ;
#46105=CARTESIAN_POINT('',(-7.,-9.,60.)) ;
#46106=CARTESIAN_POINT('',(0.,-9.,59.5)) ;
#46107=CARTESIAN_POINT('Origin',(0.,-8.5,59.5)) ;
#46108=CARTESIAN_POINT('',(-7.,-8.5,59.5)) ;
#46109=CARTESIAN_POINT('Origin',(-7.,-8.5,60.)) ;
#46110=CARTESIAN_POINT('Origin',(7.,-8.5,60.)) ;
#46111=CARTESIAN_POINT('Origin',(0.5,-8.5,52.)) ;
#46112=CARTESIAN_POINT('',(0.5,-12.5,52.5)) ;
#46113=CARTESIAN_POINT('',(0.5,-8.5,52.5)) ;
#46114=CARTESIAN_POINT('',(0.5,-12.5,51.5)) ;
#46115=CARTESIAN_POINT('',(0.5,-12.5,52.)) ;
#46116=CARTESIAN_POINT('',(0.5,-8.5,51.5)) ;
#46117=CARTESIAN_POINT('Origin',(0.,-8.5,52.5)) ;
#46118=CARTESIAN_POINT('',(-0.5,-12.5,52.5)) ;
#46119=CARTESIAN_POINT('',(-0.5,-8.5,52.5)) ;
#46120=CARTESIAN_POINT('',(-2.44929359829471E-16,-12.5,52.5)) ;
#46121=CARTESIAN_POINT('Origin',(0.,-8.5,51.5)) ;
#46122=CARTESIAN_POINT('',(-0.5,-12.5,51.5)) ;
#46123=CARTESIAN_POINT('',(-2.44929359829471E-16,-12.5,51.5)) ;
#46124=CARTESIAN_POINT('',(-0.5,-8.5,51.5)) ;
#46125=CARTESIAN_POINT('Origin',(0.,-8.5,51.5)) ;
#46126=CARTESIAN_POINT('',(-0.5,-4.5,51.5)) ;
#46127=CARTESIAN_POINT('',(-0.5,-8.5,51.5)) ;
#46128=CARTESIAN_POINT('',(0.5,-4.5,51.5)) ;
#46129=CARTESIAN_POINT('',(2.44929359829471E-16,-4.5,51.5)) ;
#46130=CARTESIAN_POINT('',(0.5,-8.5,51.5)) ;
#46131=CARTESIAN_POINT('Origin',(-0.5,-8.5,52.)) ;
#46132=CARTESIAN_POINT('',(-0.5,-12.5,52.)) ;
#46133=CARTESIAN_POINT('Origin',(-0.5,-8.5,52.)) ;
#46134=CARTESIAN_POINT('',(-0.5,-4.5,52.5)) ;
#46135=CARTESIAN_POINT('',(-0.5,-8.5,52.5)) ;
#46136=CARTESIAN_POINT('',(-0.5,-4.5,52.)) ;
#46137=CARTESIAN_POINT('Origin',(0.5,-8.5,52.)) ;
#46138=CARTESIAN_POINT('',(0.5,-4.5,52.5)) ;
#46139=CARTESIAN_POINT('',(0.5,-4.5,52.)) ;
#46140=CARTESIAN_POINT('',(0.5,-8.5,52.5)) ;
#46141=CARTESIAN_POINT('Origin',(-2.44929359829471E-16,-12.5,52.)) ;
#46142=CARTESIAN_POINT('Origin',(0.,-8.5,52.5)) ;
#46143=CARTESIAN_POINT('',(2.44929359829471E-16,-4.5,52.5)) ;
#46144=CARTESIAN_POINT('Origin',(2.44929359829471E-16,-4.5,52.)) ;
#46145=CARTESIAN_POINT('Origin',(0.,-9.,52.)) ;
#46146=CARTESIAN_POINT('',(4.,-9.,51.5)) ;
#46147=CARTESIAN_POINT('',(0.,-9.,51.5)) ;
#46148=CARTESIAN_POINT('',(4.,-9.,52.5)) ;
#46149=CARTESIAN_POINT('',(4.,-9.,52.)) ;
#46150=CARTESIAN_POINT('',(0.,-9.,52.5)) ;
#46151=CARTESIAN_POINT('Origin',(0.,-8.5,51.5)) ;
#46152=CARTESIAN_POINT('',(4.,-8.,51.5)) ;
#46153=CARTESIAN_POINT('',(0.,-8.,51.5)) ;
#46154=CARTESIAN_POINT('',(4.,-8.5,51.5)) ;
#46155=CARTESIAN_POINT('Origin',(0.,-8.5,52.5)) ;
#46156=CARTESIAN_POINT('',(4.,-8.,52.5)) ;
#46157=CARTESIAN_POINT('',(4.,-8.5,52.5)) ;
#46158=CARTESIAN_POINT('',(0.,-8.,52.5)) ;
#46159=CARTESIAN_POINT('Origin',(0.,-8.5,52.5)) ;
#46160=CARTESIAN_POINT('',(-4.,-8.,52.5)) ;
#46161=CARTESIAN_POINT('',(0.,-8.,52.5)) ;
#46162=CARTESIAN_POINT('',(-4.,-9.,52.5)) ;
#46163=CARTESIAN_POINT('',(-4.,-8.5,52.5)) ;
#46164=CARTESIAN_POINT('',(0.,-9.,52.5)) ;
#46165=CARTESIAN_POINT('Origin',(0.,-8.,52.)) ;
#46166=CARTESIAN_POINT('',(4.,-8.,52.)) ;
#46167=CARTESIAN_POINT('Origin',(0.,-8.,52.)) ;
#46168=CARTESIAN_POINT('',(-4.,-8.,51.5)) ;
#46169=CARTESIAN_POINT('',(0.,-8.,51.5)) ;
#46170=CARTESIAN_POINT('',(-4.,-8.,52.)) ;
#46171=CARTESIAN_POINT('Origin',(0.,-9.,52.)) ;
#46172=CARTESIAN_POINT('',(-4.,-9.,51.5)) ;
#46173=CARTESIAN_POINT('',(-4.,-9.,52.)) ;
#46174=CARTESIAN_POINT('',(0.,-9.,51.5)) ;
#46175=CARTESIAN_POINT('Origin',(0.,-8.5,51.5)) ;
#46176=CARTESIAN_POINT('',(-4.,-8.5,51.5)) ;
#46177=CARTESIAN_POINT('Origin',(-4.,-8.5,52.)) ;
#46178=CARTESIAN_POINT('Origin',(4.,-8.5,52.)) ;
#46179=CARTESIAN_POINT('Origin',(0.,-8.5,55.)) ;
#46180=CARTESIAN_POINT('',(-1.,-8.5,40.)) ;
#46181=CARTESIAN_POINT('',(-1.,-8.5,55.)) ;
#46182=CARTESIAN_POINT('Origin',(0.,-8.5,40.)) ;
#46183=CARTESIAN_POINT('Origin',(0.,-8.5,40.)) ;
#46184=CARTESIAN_POINT('Origin',(0.,-8.5,70.)) ;
#50356=UNCERTAINTY_MEASURE_WITH_UNIT(LENGTH_MEASURE(0.001),#50441,
'DISTANCE_ACCURACY_VALUE',
'Maximum model space distance between geometric entities at asserted c
onnectivities') ;
#50387=UNCERTAINTY_MEASURE_WITH_UNIT(LENGTH_MEASURE(0.001),#50441,
'DISTANCE_ACCURACY_VALUE',
'Maximum model space distance between geometric entities at asserted c
onnectivities') ;
#50409=(
GEOMETRIC_REPRESENTATION_CONTEXT(3)
GLOBAL_UNCERTAINTY_ASSIGNED_CONTEXT((#50356))
GLOBAL_UNIT_ASSIGNED_CONTEXT((#50441,#50443,#50444))
REPRESENTATION_CONTEXT('','3D')
) ;
#50440=(
GEOMETRIC_REPRESENTATION_CONTEXT(3)
GLOBAL_UNCERTAINTY_ASSIGNED_CONTEXT((#50387))
GLOBAL_UNIT_ASSIGNED_CONTEXT((#50441,#50443,#50444))
REPRESENTATION_CONTEXT('','3D')
) ;
#50441=(
LENGTH_UNIT()
NAMED_UNIT(*)
SI_UNIT(.CENTI.,.METRE.)
) ;
#50443=(
NAMED_UNIT(*)
PLANE_ANGLE_UNIT()
SI_UNIT($,.RADIAN.)
) ;
#50444=(
NAMED_UNIT(*)
SI_UNIT($,.STERADIAN.)
SOLID_ANGLE_UNIT()
) ;
#50466=SHAPE_DEFINITION_REPRESENTATION(#50532,#50640) ;
#50532=PRODUCT_DEFINITION_SHAPE('',$,#50693) ;
#50640=SHAPE_REPRESENTATION('',(#30580),#50409) ;
#50671=PRODUCT_DEFINITION_CONTEXT('part definition',#50829,'design') ;
#50693=PRODUCT_DEFINITION('AGITATOR_SHAFT_ASSEMBLY',
'AGITATOR_SHAFT_ASSEMBLY',#50745,#50671) ;
#50745=PRODUCT_DEFINITION_FORMATION('',$,#50852) ;
#50829=APPLICATION_CONTEXT(
'Core Data for Automotive Mechanical Design Process') ;
#50830=PRODUCT_CONTEXT('part definition',#50829,'mechanical') ;
#50852=PRODUCT('AGITATOR_SHAFT_ASSEMBLY','AGITATOR_SHAFT_ASSEMBLY',$,(#50830)) ;
#50889=PRESENTATION_STYLE_ASSIGNMENT((#50896)) ;
#50896=SURFACE_STYLE_USAGE(.BOTH.,#50903) ;
#50903=SURFACE_SIDE_STYLE('',(#50910)) ;
#50910=SURFACE_STYLE_FILL_AREA(#50917) ;
#50917=FILL_AREA_STYLE('Stainless Steel - Satin',(#50924)) ;
#50924=FILL_AREA_STYLE_COLOUR('Stainless Steel - Satin',#50931) ;
#50931=COLOUR_RGB('Stainless Steel - Satin', 0.72549020, 0.75294118, 0.79215686) ;
ENDSEC;
END-ISO-10303-21;
